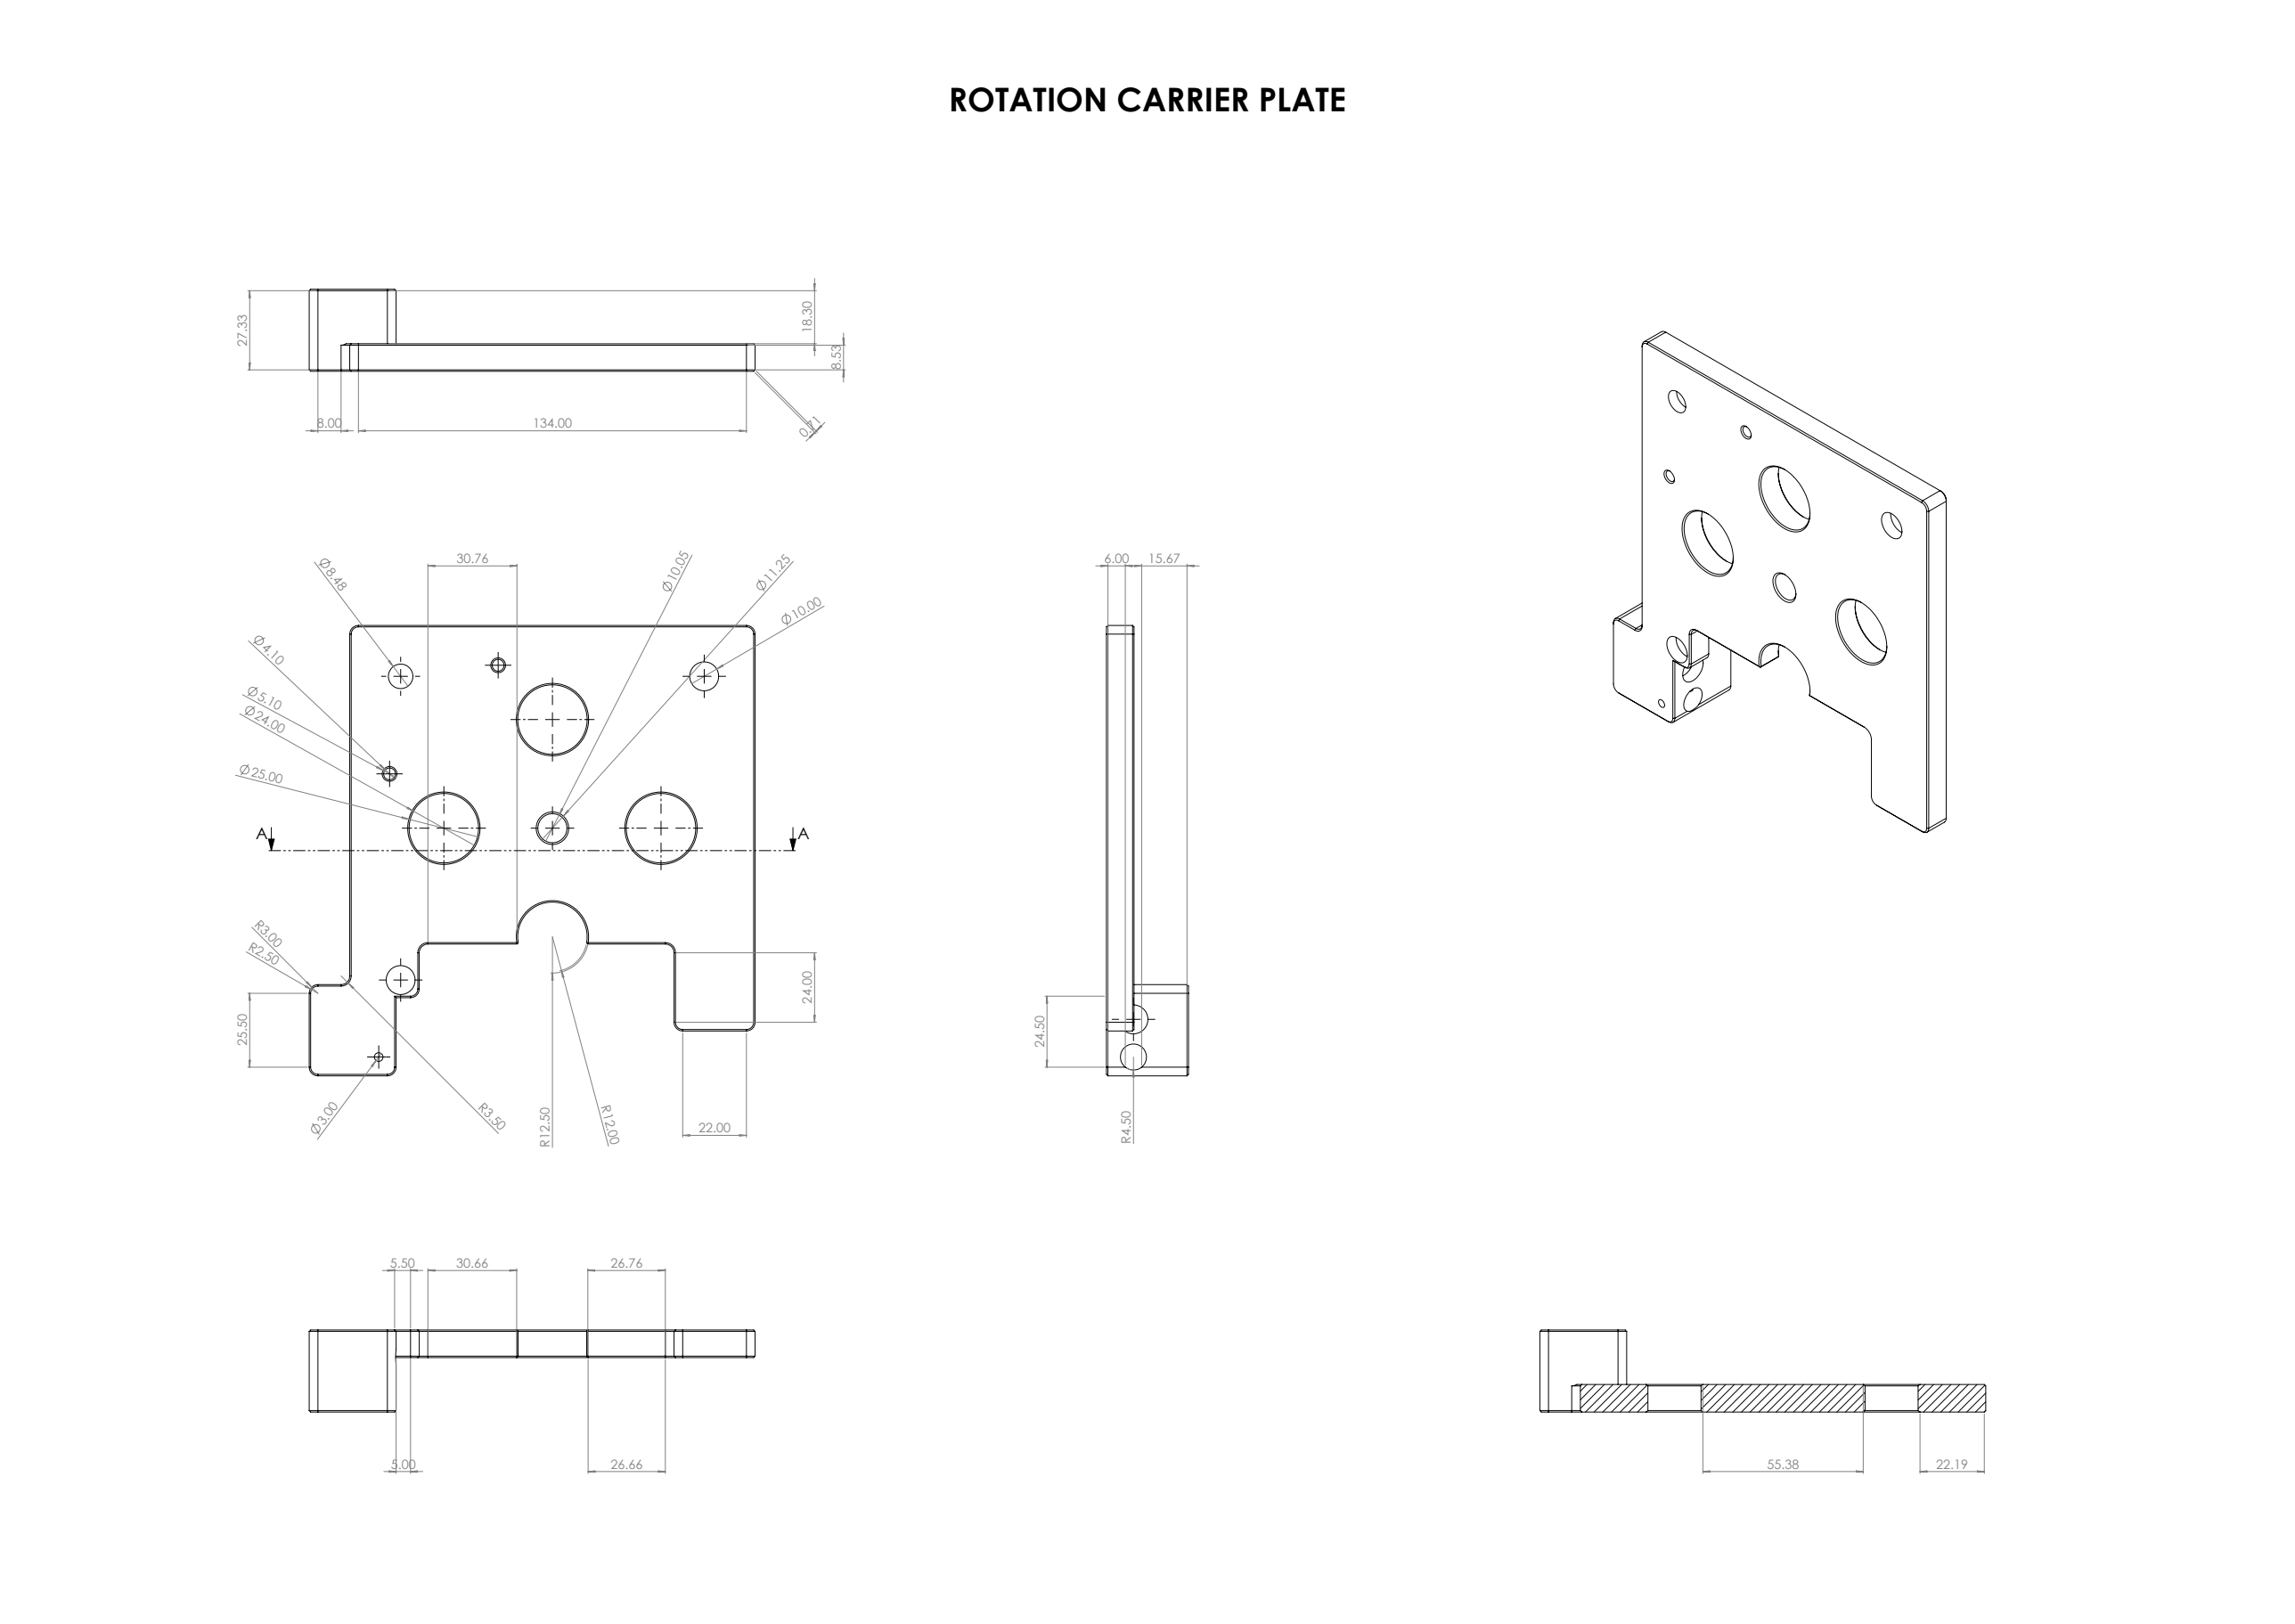
ISO-10303-21;
HEADER;
/* Generated by software containing ST-Developer
 * from STEP Tools, Inc. (www.steptools.com) 
 */

FILE_DESCRIPTION(
/* description */ (''),
/* implementation_level */ '2;1');

FILE_NAME(
/* name */ '02_Rotation_Carrier_Plate.step',
/* time_stamp */ '2026-10-21T01:56:51-07:00',
/* author */ (''),
/* organization */ (''),
/* preprocessor_version */ 'ST-DEVELOPER v20.2',
/* originating_system */ 'Autodesk Translation Framework v15.15.0.0',
/* authorisation */ '');

FILE_SCHEMA (('AUTOMOTIVE_DESIGN { 1 0 10303 214 3 1 1 }'));
ENDSEC;

DATA;
#10=MECHANICAL_DESIGN_GEOMETRIC_PRESENTATION_REPRESENTATION('',(#271),#82384);
#162=(
BOUNDED_CURVE()
B_SPLINE_CURVE(2,(#43228,#43229,#43230),.UNSPECIFIED.,.F.,.F.)
B_SPLINE_CURVE_WITH_KNOTS((3,3),(0.0459620214738357,0.0928848613146929),
 .UNSPECIFIED.)
CURVE()
GEOMETRIC_REPRESENTATION_ITEM()
RATIONAL_B_SPLINE_CURVE((1.,1.,1.))
REPRESENTATION_ITEM('')
);
#163=(
BOUNDED_CURVE()
B_SPLINE_CURVE(2,(#43236,#43237,#43238),.UNSPECIFIED.,.F.,.F.)
B_SPLINE_CURVE_WITH_KNOTS((3,3),(0.,0.040804494448543),.UNSPECIFIED.)
CURVE()
GEOMETRIC_REPRESENTATION_ITEM()
RATIONAL_B_SPLINE_CURVE((1.,1.0001754834699,1.00017645997855))
REPRESENTATION_ITEM('')
);
#164=(
BOUNDED_CURVE()
B_SPLINE_CURVE(2,(#43242,#43243,#43244),.UNSPECIFIED.,.F.,.F.)
B_SPLINE_CURVE_WITH_KNOTS((3,3),(0.0412611632307347,0.0820656576920018),
 .UNSPECIFIED.)
CURVE()
GEOMETRIC_REPRESENTATION_ITEM()
RATIONAL_B_SPLINE_CURVE((1.00017645997855,1.00017548346996,1.))
REPRESENTATION_ITEM('')
);
#165=(
BOUNDED_CURVE()
B_SPLINE_CURVE(2,(#43257,#43258,#43259),.UNSPECIFIED.,.F.,.F.)
B_SPLINE_CURVE_WITH_KNOTS((3,3),(2.77288184399903,2.88132188410877),
 .UNSPECIFIED.)
CURVE()
GEOMETRIC_REPRESENTATION_ITEM()
RATIONAL_B_SPLINE_CURVE((1.00662865875794,1.0034439439933,1.))
REPRESENTATION_ITEM('')
);
#166=(
BOUNDED_CURVE()
B_SPLINE_CURVE(2,(#43294,#43295,#43296),.UNSPECIFIED.,.F.,.F.)
B_SPLINE_CURVE_WITH_KNOTS((3,3),(0.0225541082777549,0.04593400953422),
 .UNSPECIFIED.)
CURVE()
GEOMETRIC_REPRESENTATION_ITEM()
RATIONAL_B_SPLINE_CURVE((1.01228995969815,1.01859260314039,1.02475566063204))
REPRESENTATION_ITEM('')
);
#167=(
BOUNDED_CURVE()
B_SPLINE_CURVE(2,(#43300,#43301,#43302),.UNSPECIFIED.,.F.,.F.)
B_SPLINE_CURVE_WITH_KNOTS((3,3),(0.,0.0469228395759985),.UNSPECIFIED.)
CURVE()
GEOMETRIC_REPRESENTATION_ITEM()
RATIONAL_B_SPLINE_CURVE((1.,1.,1.))
REPRESENTATION_ITEM('')
);
#168=(
BOUNDED_CURVE()
B_SPLINE_CURVE(2,(#43425,#43426,#43427),.UNSPECIFIED.,.F.,.F.)
B_SPLINE_CURVE_WITH_KNOTS((3,3),(0.188460067452875,0.376920134905751),
 .UNSPECIFIED.)
CURVE()
GEOMETRIC_REPRESENTATION_ITEM()
RATIONAL_B_SPLINE_CURVE((1.,1.04083299973288,1.))
REPRESENTATION_ITEM('')
);
#233=SHAPE_REPRESENTATION_RELATIONSHIP('SRR','None',#82467,#252);
#252=ADVANCED_BREP_SHAPE_REPRESENTATION('',(#290),#82366);
#271=STYLED_ITEM('',(#82617),#290);
#290=MANIFOLD_SOLID_BREP('Body1',#30662);
#457=CYLINDRICAL_SURFACE('',#31148,2.05);
#458=CYLINDRICAL_SURFACE('',#31152,2.05);
#459=CYLINDRICAL_SURFACE('',#31178,3.);
#460=CYLINDRICAL_SURFACE('',#31180,12.);
#461=CYLINDRICAL_SURFACE('',#31197,12.);
#462=CYLINDRICAL_SURFACE('',#31201,12.);
#463=CYLINDRICAL_SURFACE('',#31205,12.);
#464=CYLINDRICAL_SURFACE('',#31241,3.);
#465=CYLINDRICAL_SURFACE('',#31244,3.);
#466=CYLINDRICAL_SURFACE('',#31277,3.);
#467=CYLINDRICAL_SURFACE('',#31279,3.);
#468=CYLINDRICAL_SURFACE('',#31281,3.);
#469=CYLINDRICAL_SURFACE('',#31283,3.);
#470=CYLINDRICAL_SURFACE('',#31285,3.);
#471=CYLINDRICAL_SURFACE('',#31287,3.);
#472=CYLINDRICAL_SURFACE('',#31289,3.);
#473=CYLINDRICAL_SURFACE('',#31296,5.025);
#474=CYLINDRICAL_SURFACE('',#31297,1.5);
#475=CYLINDRICAL_SURFACE('',#31298,1.5);
#476=CYLINDRICAL_SURFACE('',#31301,4.5);
#477=CYLINDRICAL_SURFACE('',#31304,5.);
#478=CYLINDRICAL_SURFACE('',#31309,4.2379);
#479=CYLINDRICAL_SURFACE('',#31312,5.);
#480=CYLINDRICAL_SURFACE('',#31315,5.);
#481=CYLINDRICAL_SURFACE('',#31318,3.);
#482=CYLINDRICAL_SURFACE('',#31320,3.);
#1111=CIRCLE('',#31124,2.55);
#1112=CIRCLE('',#31125,2.05);
#1113=CIRCLE('',#31127,2.5);
#1114=CIRCLE('',#31128,3.5);
#1115=CIRCLE('',#31129,12.5);
#1116=CIRCLE('',#31130,3.5);
#1117=CIRCLE('',#31131,2.5);
#1118=CIRCLE('',#31132,2.5);
#1119=CIRCLE('',#31133,2.5);
#1120=CIRCLE('',#31134,2.5);
#1121=CIRCLE('',#31135,3.5);
#1122=CIRCLE('',#31136,2.5);
#1123=CIRCLE('',#31137,2.5);
#1124=CIRCLE('',#31138,2.50000000000001);
#1125=CIRCLE('',#31139,2.55);
#1126=CIRCLE('',#31140,12.5);
#1127=CIRCLE('',#31141,12.5);
#1128=CIRCLE('',#31142,1.5);
#1129=CIRCLE('',#31143,5.);
#1130=CIRCLE('',#31144,5.);
#1131=CIRCLE('',#31145,4.2379);
#1132=CIRCLE('',#31146,5.625);
#1133=CIRCLE('',#31147,12.5);
#1134=CIRCLE('',#31149,2.05);
#1135=CIRCLE('',#31151,2.05);
#1136=CIRCLE('',#31153,2.05);
#1137=CIRCLE('',#31156,3.);
#1138=CIRCLE('',#31159,3.);
#1139=CIRCLE('',#31162,12.);
#1140=CIRCLE('',#31167,3.);
#1141=CIRCLE('',#31168,2.5);
#1142=CIRCLE('',#31171,3.);
#1143=CIRCLE('',#31172,3.5);
#1144=CIRCLE('',#31175,12.);
#1145=CIRCLE('',#31176,12.5);
#1146=CIRCLE('',#31184,12.5);
#1147=CIRCLE('',#31185,12.);
#1148=CIRCLE('',#31187,3.);
#1149=CIRCLE('',#31188,3.5);
#1150=CIRCLE('',#31189,2.5);
#1151=CIRCLE('',#31190,2.5);
#1152=CIRCLE('',#31191,2.5);
#1153=CIRCLE('',#31192,2.5);
#1154=CIRCLE('',#31193,3.5);
#1155=CIRCLE('',#31194,12.5);
#1156=CIRCLE('',#31195,5.025);
#1157=CIRCLE('',#31196,12.5);
#1158=CIRCLE('',#31198,12.);
#1159=CIRCLE('',#31200,12.);
#1160=CIRCLE('',#31202,12.);
#1161=CIRCLE('',#31204,12.);
#1162=CIRCLE('',#31206,12.);
#1163=CIRCLE('',#31208,3.);
#1164=CIRCLE('',#31211,3.);
#1165=CIRCLE('',#31214,3.);
#1166=CIRCLE('',#31217,3.);
#1167=CIRCLE('',#31220,3.);
#1168=CIRCLE('',#31223,3.);
#1169=CIRCLE('',#31227,3.);
#1170=CIRCLE('',#31228,2.5);
#1171=CIRCLE('',#31231,3.);
#1172=CIRCLE('',#31232,2.5);
#1173=CIRCLE('',#31235,3.);
#1174=CIRCLE('',#31236,2.5);
#1175=CIRCLE('',#31239,3.);
#1176=CIRCLE('',#31240,2.50000000000001);
#1177=CIRCLE('',#31242,3.);
#1178=CIRCLE('',#31245,3.);
#1179=CIRCLE('',#31247,4.5);
#1180=CIRCLE('',#31248,4.5);
#1181=CIRCLE('',#31249,5.);
#1182=CIRCLE('',#31252,3.);
#1183=CIRCLE('',#31255,3.);
#1184=CIRCLE('',#31258,3.);
#1185=CIRCLE('',#31261,3.);
#1186=CIRCLE('',#31264,3.);
#1187=CIRCLE('',#31267,3.);
#1188=CIRCLE('',#31270,3.);
#1189=CIRCLE('',#31295,5.025);
#1190=CIRCLE('',#31299,1.5);
#1191=CIRCLE('',#31302,4.5);
#1192=CIRCLE('',#31305,5.);
#1193=CIRCLE('',#31310,4.2379);
#1194=CIRCLE('',#31313,5.);
#1195=CIRCLE('',#31316,5.);
#1899=CONICAL_SURFACE('',#31123,2.3,0.785398163397448);
#1900=CONICAL_SURFACE('',#31150,2.3,0.785398163397451);
#1901=CONICAL_SURFACE('',#31155,2.75,0.785398163397449);
#1902=CONICAL_SURFACE('',#31158,3.25,0.785398163397449);
#1903=CONICAL_SURFACE('',#31161,12.25,0.785398163397448);
#1904=CONICAL_SURFACE('',#31166,2.75,0.785398163397449);
#1905=CONICAL_SURFACE('',#31170,3.25,0.785398163397449);
#1906=CONICAL_SURFACE('',#31174,12.25,0.785398163397455);
#1907=CONICAL_SURFACE('',#31183,12.25,0.785398163397451);
#1908=CONICAL_SURFACE('',#31199,12.25,0.785398163397448);
#1909=CONICAL_SURFACE('',#31203,12.25,0.785398163397448);
#1910=CONICAL_SURFACE('',#31207,3.25,0.785398163397448);
#1911=CONICAL_SURFACE('',#31210,2.75,0.785398163397449);
#1912=CONICAL_SURFACE('',#31213,2.75,0.785398163397449);
#1913=CONICAL_SURFACE('',#31216,2.75,0.785398163397449);
#1914=CONICAL_SURFACE('',#31219,2.75,0.785398163397449);
#1915=CONICAL_SURFACE('',#31222,3.25,0.785398163397448);
#1916=CONICAL_SURFACE('',#31226,2.75,0.785398163397448);
#1917=CONICAL_SURFACE('',#31230,2.75,0.785398163397447);
#1918=CONICAL_SURFACE('',#31234,2.75,0.785398163397447);
#1919=CONICAL_SURFACE('',#31238,2.75,0.785398163397443);
#1920=CONICAL_SURFACE('',#31251,3.25,0.785398163397448);
#1921=CONICAL_SURFACE('',#31254,2.75,0.785398163397449);
#1922=CONICAL_SURFACE('',#31257,2.75,0.785398163397449);
#1923=CONICAL_SURFACE('',#31260,2.75,0.785398163397449);
#1924=CONICAL_SURFACE('',#31263,2.75,0.785398163397449);
#1925=CONICAL_SURFACE('',#31266,3.25,0.785398163397448);
#1926=CONICAL_SURFACE('',#31269,2.75,0.785398163397449);
#1927=CONICAL_SURFACE('',#31272,2.75,0.785398163397449);
#1928=CONICAL_SURFACE('',#31274,2.75,0.785398163397443);
#1929=CONICAL_SURFACE('',#31291,12.25,0.785398163397448);
#1930=CONICAL_SURFACE('',#31292,12.25,0.785398163397448);
#1931=CONICAL_SURFACE('',#31293,12.25,0.785398163397451);
#1932=CONICAL_SURFACE('',#31294,5.325,0.785398163397447);
#2303=B_SPLINE_CURVE_WITH_KNOTS('',3,(#43245,#43246,#43247,#43248),
 .UNSPECIFIED.,.F.,.F.,(4,4),(0.,0.0472495496003301),.UNSPECIFIED.);
#2304=B_SPLINE_CURVE_WITH_KNOTS('',3,(#43495,#43496,#43497,#43498,#43499,
#43500,#43501,#43502,#43503,#43504),.UNSPECIFIED.,.F.,.F.,(4,2,2,2,4),(0.495600103897638,
0.617811944958686,0.790142329574639,0.962472714190591,1.08468455525164),
 .UNSPECIFIED.);
#2305=B_SPLINE_CURVE_WITH_KNOTS('',3,(#43626,#43627,#43628,#43629,#43630,
#43631,#43632,#43633,#43634,#43635,#43636,#43637,#43638,#43639,#43640,#43641,
#43642,#43643),.UNSPECIFIED.,.F.,.F.,(4,2,2,2,2,2,2,2,4),(0.227910044047723,
0.284874338888031,0.34183863372834,0.398829360911893,0.455820088095446,
0.512810815278999,0.569801542462552,0.626765837302861,0.683730132143169),
 .UNSPECIFIED.);
#2306=B_SPLINE_CURVE_WITH_KNOTS('',3,(#43645,#43646,#43647,#43648,#43649,
#43650,#43651,#43652,#43653,#43654),.UNSPECIFIED.,.F.,.F.,(4,2,2,2,4),(0.,
0.0569907271835534,0.113981454367107,0.170945749207415,0.227910044047723),
 .UNSPECIFIED.);
#2307=B_SPLINE_CURVE_WITH_KNOTS('',3,(#43655,#43656,#43657,#43658,#43659,
#43660,#43661,#43662,#43663,#43664),.UNSPECIFIED.,.F.,.F.,(4,2,2,2,4),(0.683730132143169,
0.740694426983477,0.797658721823785,0.854649449007338,0.911640176190892),
 .UNSPECIFIED.);
#2308=B_SPLINE_CURVE_WITH_KNOTS('',3,(#43668,#43669,#43670,#43671,#43672,
#43673,#43674,#43675,#43676,#43677),.UNSPECIFIED.,.F.,.F.,(4,2,2,2,4),(0.,
0.0569907271835534,0.113981454367107,0.170945749207415,0.227910044047723),
 .UNSPECIFIED.);
#2309=B_SPLINE_CURVE_WITH_KNOTS('',3,(#43678,#43679,#43680,#43681,#43682,
#43683,#43684,#43685,#43686,#43687,#43688,#43689,#43690,#43691,#43692,#43693,
#43694,#43695,#43696,#43697,#43698,#43699,#43700,#43701,#43702,#43703),
 .UNSPECIFIED.,.F.,.F.,(4,2,2,2,2,2,2,2,2,2,2,2,4),(0.227910044047723,0.284874338888031,
0.34183863372834,0.398829360911893,0.455820088095446,0.512810815278999,
0.569801542462552,0.626765837302861,0.683730132143169,0.740694426983477,
0.797658721823785,0.854649449007338,0.911640176190892),.UNSPECIFIED.);
#3321=FACE_BOUND('',#5637,.T.);
#3322=FACE_BOUND('',#5638,.T.);
#3323=FACE_BOUND('',#5639,.T.);
#3324=FACE_BOUND('',#5640,.T.);
#3325=FACE_BOUND('',#5641,.T.);
#3326=FACE_BOUND('',#5642,.T.);
#3327=FACE_BOUND('',#5643,.T.);
#3328=FACE_BOUND('',#5644,.T.);
#3329=FACE_BOUND('',#5645,.T.);
#3330=FACE_BOUND('',#5646,.T.);
#3331=FACE_BOUND('',#5672,.T.);
#3332=FACE_BOUND('',#5673,.T.);
#3333=FACE_BOUND('',#5674,.T.);
#3334=FACE_BOUND('',#5675,.T.);
#3335=FACE_BOUND('',#5705,.T.);
#3336=FACE_BOUND('',#5749,.T.);
#3842=FACE_OUTER_BOUND('',#5635,.T.);
#3843=FACE_OUTER_BOUND('',#5636,.T.);
#3844=FACE_OUTER_BOUND('',#5647,.T.);
#3845=FACE_OUTER_BOUND('',#5648,.T.);
#3846=FACE_OUTER_BOUND('',#5649,.T.);
#3847=FACE_OUTER_BOUND('',#5650,.T.);
#3848=FACE_OUTER_BOUND('',#5651,.T.);
#3849=FACE_OUTER_BOUND('',#5652,.T.);
#3850=FACE_OUTER_BOUND('',#5653,.T.);
#3851=FACE_OUTER_BOUND('',#5654,.T.);
#3852=FACE_OUTER_BOUND('',#5655,.T.);
#3853=FACE_OUTER_BOUND('',#5656,.T.);
#3854=FACE_OUTER_BOUND('',#5657,.T.);
#3855=FACE_OUTER_BOUND('',#5658,.T.);
#3856=FACE_OUTER_BOUND('',#5659,.T.);
#3857=FACE_OUTER_BOUND('',#5660,.T.);
#3858=FACE_OUTER_BOUND('',#5661,.T.);
#3859=FACE_OUTER_BOUND('',#5662,.T.);
#3860=FACE_OUTER_BOUND('',#5663,.T.);
#3861=FACE_OUTER_BOUND('',#5664,.T.);
#3862=FACE_OUTER_BOUND('',#5665,.T.);
#3863=FACE_OUTER_BOUND('',#5666,.T.);
#3864=FACE_OUTER_BOUND('',#5667,.T.);
#3865=FACE_OUTER_BOUND('',#5668,.T.);
#3866=FACE_OUTER_BOUND('',#5669,.T.);
#3867=FACE_OUTER_BOUND('',#5670,.T.);
#3868=FACE_OUTER_BOUND('',#5671,.T.);
#3869=FACE_OUTER_BOUND('',#5676,.T.);
#3870=FACE_OUTER_BOUND('',#5677,.T.);
#3871=FACE_OUTER_BOUND('',#5678,.T.);
#3872=FACE_OUTER_BOUND('',#5679,.T.);
#3873=FACE_OUTER_BOUND('',#5680,.T.);
#3874=FACE_OUTER_BOUND('',#5681,.T.);
#3875=FACE_OUTER_BOUND('',#5682,.T.);
#3876=FACE_OUTER_BOUND('',#5683,.T.);
#3877=FACE_OUTER_BOUND('',#5684,.T.);
#3878=FACE_OUTER_BOUND('',#5685,.T.);
#3879=FACE_OUTER_BOUND('',#5686,.T.);
#3880=FACE_OUTER_BOUND('',#5687,.T.);
#3881=FACE_OUTER_BOUND('',#5688,.T.);
#3882=FACE_OUTER_BOUND('',#5689,.T.);
#3883=FACE_OUTER_BOUND('',#5690,.T.);
#3884=FACE_OUTER_BOUND('',#5691,.T.);
#3885=FACE_OUTER_BOUND('',#5692,.T.);
#3886=FACE_OUTER_BOUND('',#5693,.T.);
#3887=FACE_OUTER_BOUND('',#5694,.T.);
#3888=FACE_OUTER_BOUND('',#5695,.T.);
#3889=FACE_OUTER_BOUND('',#5696,.T.);
#3890=FACE_OUTER_BOUND('',#5697,.T.);
#3891=FACE_OUTER_BOUND('',#5698,.T.);
#3892=FACE_OUTER_BOUND('',#5699,.T.);
#3893=FACE_OUTER_BOUND('',#5700,.T.);
#3894=FACE_OUTER_BOUND('',#5701,.T.);
#3895=FACE_OUTER_BOUND('',#5702,.T.);
#3896=FACE_OUTER_BOUND('',#5703,.T.);
#3897=FACE_OUTER_BOUND('',#5704,.T.);
#3898=FACE_OUTER_BOUND('',#5706,.T.);
#3899=FACE_OUTER_BOUND('',#5707,.T.);
#3900=FACE_OUTER_BOUND('',#5708,.T.);
#3901=FACE_OUTER_BOUND('',#5709,.T.);
#3902=FACE_OUTER_BOUND('',#5710,.T.);
#3903=FACE_OUTER_BOUND('',#5711,.T.);
#3904=FACE_OUTER_BOUND('',#5712,.T.);
#3905=FACE_OUTER_BOUND('',#5713,.T.);
#3906=FACE_OUTER_BOUND('',#5714,.T.);
#3907=FACE_OUTER_BOUND('',#5715,.T.);
#3908=FACE_OUTER_BOUND('',#5716,.T.);
#3909=FACE_OUTER_BOUND('',#5717,.T.);
#3910=FACE_OUTER_BOUND('',#5718,.T.);
#3911=FACE_OUTER_BOUND('',#5719,.T.);
#3912=FACE_OUTER_BOUND('',#5720,.T.);
#3913=FACE_OUTER_BOUND('',#5721,.T.);
#3914=FACE_OUTER_BOUND('',#5722,.T.);
#3915=FACE_OUTER_BOUND('',#5723,.T.);
#3916=FACE_OUTER_BOUND('',#5724,.T.);
#3917=FACE_OUTER_BOUND('',#5725,.T.);
#3918=FACE_OUTER_BOUND('',#5726,.T.);
#3919=FACE_OUTER_BOUND('',#5727,.T.);
#3920=FACE_OUTER_BOUND('',#5728,.T.);
#3921=FACE_OUTER_BOUND('',#5729,.T.);
#3922=FACE_OUTER_BOUND('',#5730,.T.);
#3923=FACE_OUTER_BOUND('',#5731,.T.);
#3924=FACE_OUTER_BOUND('',#5732,.T.);
#3925=FACE_OUTER_BOUND('',#5733,.T.);
#3926=FACE_OUTER_BOUND('',#5734,.T.);
#3927=FACE_OUTER_BOUND('',#5735,.T.);
#3928=FACE_OUTER_BOUND('',#5736,.T.);
#3929=FACE_OUTER_BOUND('',#5737,.T.);
#3930=FACE_OUTER_BOUND('',#5738,.T.);
#3931=FACE_OUTER_BOUND('',#5739,.T.);
#3932=FACE_OUTER_BOUND('',#5740,.T.);
#3933=FACE_OUTER_BOUND('',#5741,.T.);
#3934=FACE_OUTER_BOUND('',#5742,.T.);
#3935=FACE_OUTER_BOUND('',#5743,.T.);
#3936=FACE_OUTER_BOUND('',#5744,.T.);
#3937=FACE_OUTER_BOUND('',#5745,.T.);
#3938=FACE_OUTER_BOUND('',#5746,.T.);
#3939=FACE_OUTER_BOUND('',#5747,.T.);
#3940=FACE_OUTER_BOUND('',#5748,.T.);
#3941=FACE_OUTER_BOUND('',#5750,.T.);
#3942=FACE_OUTER_BOUND('',#5751,.T.);
#3943=FACE_OUTER_BOUND('',#5752,.T.);
#3944=FACE_OUTER_BOUND('',#5753,.T.);
#3945=FACE_OUTER_BOUND('',#5754,.T.);
#3946=FACE_OUTER_BOUND('',#5755,.T.);
#3947=FACE_OUTER_BOUND('',#5756,.T.);
#3948=FACE_OUTER_BOUND('',#5757,.T.);
#3949=FACE_OUTER_BOUND('',#5758,.T.);
#3950=FACE_OUTER_BOUND('',#5759,.T.);
#3951=FACE_OUTER_BOUND('',#5760,.T.);
#3952=FACE_OUTER_BOUND('',#5761,.T.);
#3953=FACE_OUTER_BOUND('',#5762,.T.);
#3954=FACE_OUTER_BOUND('',#5763,.T.);
#5635=EDGE_LOOP('',(#20603,#20604,#20605,#20606));
#5636=EDGE_LOOP('',(#20607,#20608,#20609,#20610,#20611,#20612,#20613,#20614,
#20615,#20616,#20617,#20618,#20619,#20620,#20621,#20622,#20623,#20624,#20625,
#20626,#20627,#20628,#20629,#20630,#20631));
#5637=EDGE_LOOP('',(#20632));
#5638=EDGE_LOOP('',(#20633));
#5639=EDGE_LOOP('',(#20634));
#5640=EDGE_LOOP('',(#20635));
#5641=EDGE_LOOP('',(#20636));
#5642=EDGE_LOOP('',(#20637));
#5643=EDGE_LOOP('',(#20638));
#5644=EDGE_LOOP('',(#20639));
#5645=EDGE_LOOP('',(#20640));
#5646=EDGE_LOOP('',(#20641));
#5647=EDGE_LOOP('',(#20642,#20643,#20644,#20645));
#5648=EDGE_LOOP('',(#20646,#20647,#20648,#20649));
#5649=EDGE_LOOP('',(#20650,#20651,#20652,#20653));
#5650=EDGE_LOOP('',(#20654,#20655,#20656,#20657));
#5651=EDGE_LOOP('',(#20658,#20659,#20660,#20661));
#5652=EDGE_LOOP('',(#20662,#20663,#20664,#20665));
#5653=EDGE_LOOP('',(#20666,#20667,#20668,#20669));
#5654=EDGE_LOOP('',(#20670,#20671,#20672,#20673,#20674));
#5655=EDGE_LOOP('',(#20675,#20676,#20677,#20678,#20679,#20680));
#5656=EDGE_LOOP('',(#20681,#20682,#20683,#20684,#20685));
#5657=EDGE_LOOP('',(#20686,#20687,#20688));
#5658=EDGE_LOOP('',(#20689,#20690,#20691,#20692));
#5659=EDGE_LOOP('',(#20693,#20694,#20695,#20696));
#5660=EDGE_LOOP('',(#20697,#20698,#20699,#20700));
#5661=EDGE_LOOP('',(#20701,#20702,#20703,#20704));
#5662=EDGE_LOOP('',(#20705,#20706,#20707,#20708));
#5663=EDGE_LOOP('',(#20709,#20710,#20711,#20712,#20713));
#5664=EDGE_LOOP('',(#20714,#20715,#20716,#20717));
#5665=EDGE_LOOP('',(#20718,#20719,#20720,#20721));
#5666=EDGE_LOOP('',(#20722,#20723,#20724,#20725));
#5667=EDGE_LOOP('',(#20726,#20727,#20728,#20729));
#5668=EDGE_LOOP('',(#20730,#20731,#20732,#20733,#20734,#20735));
#5669=EDGE_LOOP('',(#20736,#20737,#20738,#20739,#20740));
#5670=EDGE_LOOP('',(#20741,#20742,#20743,#20744));
#5671=EDGE_LOOP('',(#20745,#20746,#20747,#20748,#20749,#20750,#20751,#20752,
#20753,#20754,#20755,#20756,#20757,#20758,#20759,#20760,#20761,#20762,#20763,
#20764,#20765));
#5672=EDGE_LOOP('',(#20766));
#5673=EDGE_LOOP('',(#20767));
#5674=EDGE_LOOP('',(#20768));
#5675=EDGE_LOOP('',(#20769));
#5676=EDGE_LOOP('',(#20770,#20771,#20772,#20773));
#5677=EDGE_LOOP('',(#20774,#20775,#20776,#20777));
#5678=EDGE_LOOP('',(#20778,#20779,#20780,#20781));
#5679=EDGE_LOOP('',(#20782,#20783,#20784,#20785));
#5680=EDGE_LOOP('',(#20786,#20787,#20788,#20789));
#5681=EDGE_LOOP('',(#20790,#20791,#20792,#20793));
#5682=EDGE_LOOP('',(#20794,#20795,#20796,#20797));
#5683=EDGE_LOOP('',(#20798,#20799,#20800,#20801));
#5684=EDGE_LOOP('',(#20802,#20803,#20804,#20805));
#5685=EDGE_LOOP('',(#20806,#20807,#20808,#20809));
#5686=EDGE_LOOP('',(#20810,#20811,#20812,#20813));
#5687=EDGE_LOOP('',(#20814,#20815,#20816,#20817));
#5688=EDGE_LOOP('',(#20818,#20819,#20820,#20821));
#5689=EDGE_LOOP('',(#20822,#20823,#20824,#20825));
#5690=EDGE_LOOP('',(#20826,#20827,#20828,#20829));
#5691=EDGE_LOOP('',(#20830,#20831,#20832,#20833));
#5692=EDGE_LOOP('',(#20834,#20835,#20836,#20837,#20838));
#5693=EDGE_LOOP('',(#20839,#20840,#20841,#20842));
#5694=EDGE_LOOP('',(#20843,#20844,#20845,#20846));
#5695=EDGE_LOOP('',(#20847,#20848,#20849,#20850));
#5696=EDGE_LOOP('',(#20851,#20852,#20853,#20854));
#5697=EDGE_LOOP('',(#20855,#20856,#20857,#20858));
#5698=EDGE_LOOP('',(#20859,#20860,#20861,#20862));
#5699=EDGE_LOOP('',(#20863,#20864,#20865,#20866));
#5700=EDGE_LOOP('',(#20867,#20868,#20869,#20870));
#5701=EDGE_LOOP('',(#20871,#20872,#20873,#20874));
#5702=EDGE_LOOP('',(#20875,#20876,#20877,#20878));
#5703=EDGE_LOOP('',(#20879,#20880,#20881,#20882,#20883,#20884));
#5704=EDGE_LOOP('',(#20885,#20886,#20887,#20888,#20889,#20890,#20891,#20892,
#20893,#20894));
#5705=EDGE_LOOP('',(#20895));
#5706=EDGE_LOOP('',(#20896,#20897,#20898,#20899,#20900,#20901,#20902,#20903));
#5707=EDGE_LOOP('',(#20904,#20905,#20906,#20907));
#5708=EDGE_LOOP('',(#20908,#20909,#20910,#20911));
#5709=EDGE_LOOP('',(#20912,#20913,#20914,#20915));
#5710=EDGE_LOOP('',(#20916,#20917,#20918,#20919));
#5711=EDGE_LOOP('',(#20920,#20921,#20922,#20923));
#5712=EDGE_LOOP('',(#20924,#20925,#20926,#20927));
#5713=EDGE_LOOP('',(#20928,#20929,#20930,#20931));
#5714=EDGE_LOOP('',(#20932,#20933,#20934,#20935));
#5715=EDGE_LOOP('',(#20936,#20937,#20938,#20939));
#5716=EDGE_LOOP('',(#20940,#20941,#20942,#20943));
#5717=EDGE_LOOP('',(#20944,#20945,#20946,#20947));
#5718=EDGE_LOOP('',(#20948,#20949,#20950,#20951));
#5719=EDGE_LOOP('',(#20952,#20953,#20954,#20955));
#5720=EDGE_LOOP('',(#20956,#20957,#20958,#20959));
#5721=EDGE_LOOP('',(#20960,#20961,#20962,#20963));
#5722=EDGE_LOOP('',(#20964,#20965,#20966,#20967));
#5723=EDGE_LOOP('',(#20968,#20969,#20970,#20971));
#5724=EDGE_LOOP('',(#20972,#20973,#20974,#20975));
#5725=EDGE_LOOP('',(#20976,#20977,#20978,#20979));
#5726=EDGE_LOOP('',(#20980,#20981,#20982,#20983));
#5727=EDGE_LOOP('',(#20984,#20985,#20986,#20987,#20988,#20989,#20990));
#5728=EDGE_LOOP('',(#20991,#20992,#20993,#20994));
#5729=EDGE_LOOP('',(#20995,#20996,#20997,#20998));
#5730=EDGE_LOOP('',(#20999,#21000,#21001,#21002));
#5731=EDGE_LOOP('',(#21003,#21004,#21005,#21006));
#5732=EDGE_LOOP('',(#21007,#21008,#21009,#21010));
#5733=EDGE_LOOP('',(#21011,#21012,#21013,#21014));
#5734=EDGE_LOOP('',(#21015,#21016,#21017,#21018));
#5735=EDGE_LOOP('',(#21019,#21020,#21021,#21022));
#5736=EDGE_LOOP('',(#21023,#21024,#21025,#21026));
#5737=EDGE_LOOP('',(#21027,#21028,#21029,#21030));
#5738=EDGE_LOOP('',(#21031,#21032,#21033,#21034));
#5739=EDGE_LOOP('',(#21035,#21036,#21037,#21038));
#5740=EDGE_LOOP('',(#21039,#21040,#21041,#21042));
#5741=EDGE_LOOP('',(#21043,#21044,#21045,#21046));
#5742=EDGE_LOOP('',(#21047,#21048,#21049,#21050));
#5743=EDGE_LOOP('',(#21051,#21052,#21053,#21054));
#5744=EDGE_LOOP('',(#21055,#21056,#21057,#21058));
#5745=EDGE_LOOP('',(#21059,#21060,#21061,#21062,#21063,#21064));
#5746=EDGE_LOOP('',(#21065,#21066,#21067,#21068,#21069));
#5747=EDGE_LOOP('',(#21070));
#5748=EDGE_LOOP('',(#21071,#21072,#21073,#21074,#21075,#21076,#21077,#21078,
#21079,#21080,#21081));
#5749=EDGE_LOOP('',(#21082,#21083));
#5750=EDGE_LOOP('',(#21084));
#5751=EDGE_LOOP('',(#21085,#21086,#21087,#21088));
#5752=EDGE_LOOP('',(#21089));
#5753=EDGE_LOOP('',(#21090));
#5754=EDGE_LOOP('',(#21091));
#5755=EDGE_LOOP('',(#21092,#21093,#21094,#21095));
#5756=EDGE_LOOP('',(#21096));
#5757=EDGE_LOOP('',(#21097,#21098,#21099,#21100));
#5758=EDGE_LOOP('',(#21101));
#5759=EDGE_LOOP('',(#21102,#21103,#21104,#21105));
#5760=EDGE_LOOP('',(#21106));
#5761=EDGE_LOOP('',(#21107,#21108,#21109,#21110));
#5762=EDGE_LOOP('',(#21111,#21112,#21113,#21114));
#5763=EDGE_LOOP('',(#21115,#21116,#21117,#21118));
#7754=LINE('',#43125,#10060);
#7755=LINE('',#43130,#10061);
#7756=LINE('',#43132,#10062);
#7757=LINE('',#43136,#10063);
#7758=LINE('',#43140,#10064);
#7759=LINE('',#43144,#10065);
#7760=LINE('',#43148,#10066);
#7761=LINE('',#43152,#10067);
#7762=LINE('',#43156,#10068);
#7763=LINE('',#43160,#10069);
#7764=LINE('',#43164,#10070);
#7765=LINE('',#43168,#10071);
#7766=LINE('',#43172,#10072);
#7767=LINE('',#43176,#10073);
#7768=LINE('',#43198,#10074);
#7769=LINE('',#43202,#10075);
#7770=LINE('',#43206,#10076);
#7771=LINE('',#43210,#10077);
#7772=LINE('',#43212,#10078);
#7773=LINE('',#43213,#10079);
#7774=LINE('',#43217,#10080);
#7775=LINE('',#43220,#10081);
#7776=LINE('',#43221,#10082);
#7777=LINE('',#43225,#10083);
#7778=LINE('',#43232,#10084);
#7779=LINE('',#43233,#10085);
#7780=LINE('',#43251,#10086);
#7781=LINE('',#43253,#10087);
#7782=LINE('',#43254,#10088);
#7783=LINE('',#43260,#10089);
#7784=LINE('',#43264,#10090);
#7785=LINE('',#43266,#10091);
#7786=LINE('',#43268,#10092);
#7787=LINE('',#43269,#10093);
#7788=LINE('',#43273,#10094);
#7789=LINE('',#43279,#10095);
#7790=LINE('',#43280,#10096);
#7791=LINE('',#43281,#10097);
#7792=LINE('',#43285,#10098);
#7793=LINE('',#43289,#10099);
#7794=LINE('',#43290,#10100);
#7795=LINE('',#43304,#10101);
#7796=LINE('',#43305,#10102);
#7797=LINE('',#43307,#10103);
#7798=LINE('',#43310,#10104);
#7799=LINE('',#43313,#10105);
#7800=LINE('',#43315,#10106);
#7801=LINE('',#43316,#10107);
#7802=LINE('',#43319,#10108);
#7803=LINE('',#43321,#10109);
#7804=LINE('',#43322,#10110);
#7805=LINE('',#43327,#10111);
#7806=LINE('',#43331,#10112);
#7807=LINE('',#43335,#10113);
#7808=LINE('',#43339,#10114);
#7809=LINE('',#43343,#10115);
#7810=LINE('',#43347,#10116);
#7811=LINE('',#43351,#10117);
#7812=LINE('',#43355,#10118);
#7813=LINE('',#43366,#10119);
#7814=LINE('',#43369,#10120);
#7815=LINE('',#43374,#10121);
#7816=LINE('',#43377,#10122);
#7817=LINE('',#43382,#10123);
#7818=LINE('',#43385,#10124);
#7819=LINE('',#43389,#10125);
#7820=LINE('',#43390,#10126);
#7821=LINE('',#43393,#10127);
#7822=LINE('',#43397,#10128);
#7823=LINE('',#43398,#10129);
#7824=LINE('',#43401,#10130);
#7825=LINE('',#43405,#10131);
#7826=LINE('',#43406,#10132);
#7827=LINE('',#43409,#10133);
#7828=LINE('',#43413,#10134);
#7829=LINE('',#43414,#10135);
#7830=LINE('',#43417,#10136);
#7831=LINE('',#43421,#10137);
#7832=LINE('',#43422,#10138);
#7833=LINE('',#43431,#10139);
#7834=LINE('',#43432,#10140);
#7835=LINE('',#43436,#10141);
#7836=LINE('',#43438,#10142);
#7837=LINE('',#43440,#10143);
#7838=LINE('',#43441,#10144);
#7839=LINE('',#43445,#10145);
#7840=LINE('',#43451,#10146);
#7841=LINE('',#43452,#10147);
#7842=LINE('',#43453,#10148);
#7843=LINE('',#43457,#10149);
#7844=LINE('',#43463,#10150);
#7845=LINE('',#43464,#10151);
#7846=LINE('',#43465,#10152);
#7847=LINE('',#43469,#10153);
#7848=LINE('',#43475,#10154);
#7849=LINE('',#43476,#10155);
#7850=LINE('',#43477,#10156);
#7851=LINE('',#43483,#10157);
#7852=LINE('',#43486,#10158);
#7853=LINE('',#43489,#10159);
#7854=LINE('',#43490,#10160);
#7855=LINE('',#43493,#10161);
#7856=LINE('',#43506,#10162);
#7857=LINE('',#43509,#10163);
#7858=LINE('',#43510,#10164);
#7859=LINE('',#43511,#10165);
#7860=LINE('',#43521,#10166);
#7861=LINE('',#43524,#10167);
#7862=LINE('',#43525,#10168);
#7863=LINE('',#43529,#10169);
#7864=LINE('',#43532,#10170);
#7865=LINE('',#43533,#10171);
#7866=LINE('',#43537,#10172);
#7867=LINE('',#43540,#10173);
#7868=LINE('',#43541,#10174);
#7869=LINE('',#43545,#10175);
#7870=LINE('',#43548,#10176);
#7871=LINE('',#43549,#10177);
#7872=LINE('',#43553,#10178);
#7873=LINE('',#43556,#10179);
#7874=LINE('',#43557,#10180);
#7875=LINE('',#43561,#10181);
#7876=LINE('',#43564,#10182);
#7877=LINE('',#43565,#10183);
#7878=LINE('',#43569,#10184);
#7879=LINE('',#43571,#10185);
#7880=LINE('',#43572,#10186);
#7881=LINE('',#43574,#10187);
#7882=LINE('',#43576,#10188);
#7883=LINE('',#43578,#10189);
#7884=LINE('',#43581,#10190);
#7885=LINE('',#43583,#10191);
#7886=LINE('',#43585,#10192);
#7887=LINE('',#43586,#10193);
#7888=LINE('',#43588,#10194);
#7889=LINE('',#43590,#10195);
#7890=LINE('',#43592,#10196);
#7891=LINE('',#43594,#10197);
#7892=LINE('',#43596,#10198);
#7893=LINE('',#43598,#10199);
#7894=LINE('',#43600,#10200);
#7895=LINE('',#43602,#10201);
#7896=LINE('',#43604,#10202);
#7897=LINE('',#43606,#10203);
#7898=LINE('',#43608,#10204);
#7899=LINE('',#43611,#10205);
#7900=LINE('',#43613,#10206);
#7901=LINE('',#43615,#10207);
#7902=LINE('',#43618,#10208);
#7903=LINE('',#43621,#10209);
#7904=LINE('',#43624,#10210);
#7905=LINE('',#43705,#10211);
#7906=LINE('',#43709,#10212);
#7907=LINE('',#43711,#10213);
#7908=LINE('',#43716,#10214);
#7909=LINE('',#43723,#10215);
#7910=LINE('',#43728,#10216);
#7911=LINE('',#43733,#10217);
#7912=LINE('',#43737,#10218);
#10060=VECTOR('',#34255,2.3);
#10061=VECTOR('',#34260,10.);
#10062=VECTOR('',#34261,10.);
#10063=VECTOR('',#34264,10.);
#10064=VECTOR('',#34267,10.);
#10065=VECTOR('',#34270,10.);
#10066=VECTOR('',#34273,10.);
#10067=VECTOR('',#34276,10.);
#10068=VECTOR('',#34279,10.);
#10069=VECTOR('',#34282,10.);
#10070=VECTOR('',#34285,10.);
#10071=VECTOR('',#34288,10.);
#10072=VECTOR('',#34291,10.);
#10073=VECTOR('',#34294,10.);
#10074=VECTOR('',#34317,2.05);
#10075=VECTOR('',#34322,2.3);
#10076=VECTOR('',#34327,2.05);
#10077=VECTOR('',#34332,10.);
#10078=VECTOR('',#34333,10.);
#10079=VECTOR('',#34334,10.);
#10080=VECTOR('',#34339,10.);
#10081=VECTOR('',#34342,10.);
#10082=VECTOR('',#34343,10.);
#10083=VECTOR('',#34348,10.);
#10084=VECTOR('',#34351,10.);
#10085=VECTOR('',#34352,10.);
#10086=VECTOR('',#34359,10.);
#10087=VECTOR('',#34360,10.);
#10088=VECTOR('',#34361,10.);
#10089=VECTOR('',#34364,10.);
#10090=VECTOR('',#34367,10.);
#10091=VECTOR('',#34368,10.);
#10092=VECTOR('',#34369,10.);
#10093=VECTOR('',#34370,10.);
#10094=VECTOR('',#34373,10.);
#10095=VECTOR('',#34380,10.);
#10096=VECTOR('',#34381,10.);
#10097=VECTOR('',#34382,10.);
#10098=VECTOR('',#34385,10.);
#10099=VECTOR('',#34392,10.);
#10100=VECTOR('',#34393,10.);
#10101=VECTOR('',#34402,10.);
#10102=VECTOR('',#34403,10.);
#10103=VECTOR('',#34406,10.);
#10104=VECTOR('',#34411,10.);
#10105=VECTOR('',#34414,10.);
#10106=VECTOR('',#34415,10.);
#10107=VECTOR('',#34416,10.);
#10108=VECTOR('',#34419,10.);
#10109=VECTOR('',#34420,10.);
#10110=VECTOR('',#34421,10.);
#10111=VECTOR('',#34426,12.25);
#10112=VECTOR('',#34431,10.);
#10113=VECTOR('',#34434,10.);
#10114=VECTOR('',#34437,10.);
#10115=VECTOR('',#34440,10.);
#10116=VECTOR('',#34443,10.);
#10117=VECTOR('',#34446,10.);
#10118=VECTOR('',#34449,10.);
#10119=VECTOR('',#34462,12.);
#10120=VECTOR('',#34465,12.25);
#10121=VECTOR('',#34472,12.);
#10122=VECTOR('',#34475,12.25);
#10123=VECTOR('',#34482,12.);
#10124=VECTOR('',#34485,10.);
#10125=VECTOR('',#34490,10.);
#10126=VECTOR('',#34491,10.);
#10127=VECTOR('',#34494,10.);
#10128=VECTOR('',#34499,10.);
#10129=VECTOR('',#34500,10.);
#10130=VECTOR('',#34503,10.);
#10131=VECTOR('',#34508,10.);
#10132=VECTOR('',#34509,10.);
#10133=VECTOR('',#34512,10.);
#10134=VECTOR('',#34517,10.);
#10135=VECTOR('',#34518,10.);
#10136=VECTOR('',#34521,10.);
#10137=VECTOR('',#34526,10.);
#10138=VECTOR('',#34527,10.);
#10139=VECTOR('',#34534,10.);
#10140=VECTOR('',#34535,10.);
#10141=VECTOR('',#34538,10.);
#10142=VECTOR('',#34539,10.);
#10143=VECTOR('',#34540,10.);
#10144=VECTOR('',#34541,10.);
#10145=VECTOR('',#34544,10.);
#10146=VECTOR('',#34551,10.);
#10147=VECTOR('',#34552,10.);
#10148=VECTOR('',#34553,10.);
#10149=VECTOR('',#34556,10.);
#10150=VECTOR('',#34563,10.);
#10151=VECTOR('',#34564,10.);
#10152=VECTOR('',#34565,10.);
#10153=VECTOR('',#34568,10.);
#10154=VECTOR('',#34575,10.);
#10155=VECTOR('',#34576,10.);
#10156=VECTOR('',#34577,10.);
#10157=VECTOR('',#34586,10.);
#10158=VECTOR('',#34589,10.);
#10159=VECTOR('',#34592,10.);
#10160=VECTOR('',#34593,10.);
#10161=VECTOR('',#34596,10.);
#10162=VECTOR('',#34597,10.);
#10163=VECTOR('',#34602,10.);
#10164=VECTOR('',#34603,10.);
#10165=VECTOR('',#34604,10.);
#10166=VECTOR('',#34617,10.);
#10167=VECTOR('',#34620,10.);
#10168=VECTOR('',#34621,10.);
#10169=VECTOR('',#34626,10.);
#10170=VECTOR('',#34629,10.);
#10171=VECTOR('',#34630,10.);
#10172=VECTOR('',#34635,10.);
#10173=VECTOR('',#34638,10.);
#10174=VECTOR('',#34639,10.);
#10175=VECTOR('',#34644,10.);
#10176=VECTOR('',#34647,10.);
#10177=VECTOR('',#34648,10.);
#10178=VECTOR('',#34653,10.);
#10179=VECTOR('',#34656,10.);
#10180=VECTOR('',#34657,10.);
#10181=VECTOR('',#34662,10.);
#10182=VECTOR('',#34665,10.);
#10183=VECTOR('',#34666,10.);
#10184=VECTOR('',#34671,10.);
#10185=VECTOR('',#34674,10.);
#10186=VECTOR('',#34675,10.);
#10187=VECTOR('',#34678,10.);
#10188=VECTOR('',#34681,10.);
#10189=VECTOR('',#34684,10.);
#10190=VECTOR('',#34689,10.);
#10191=VECTOR('',#34692,10.);
#10192=VECTOR('',#34695,10.);
#10193=VECTOR('',#34696,10.);
#10194=VECTOR('',#34699,10.);
#10195=VECTOR('',#34702,10.);
#10196=VECTOR('',#34705,10.);
#10197=VECTOR('',#34708,10.);
#10198=VECTOR('',#34711,10.);
#10199=VECTOR('',#34714,10.);
#10200=VECTOR('',#34717,10.);
#10201=VECTOR('',#34720,10.);
#10202=VECTOR('',#34723,10.);
#10203=VECTOR('',#34726,10.);
#10204=VECTOR('',#34729,10.);
#10205=VECTOR('',#34734,12.25);
#10206=VECTOR('',#34737,12.25);
#10207=VECTOR('',#34740,12.25);
#10208=VECTOR('',#34743,5.325);
#10209=VECTOR('',#34748,5.025);
#10210=VECTOR('',#34751,1.5);
#10211=VECTOR('',#34754,1.5);
#10212=VECTOR('',#34761,4.5);
#10213=VECTOR('',#34762,4.5);
#10214=VECTOR('',#34769,5.);
#10215=VECTOR('',#34780,4.2379);
#10216=VECTOR('',#34787,5.);
#10217=VECTOR('',#34794,5.);
#10218=VECTOR('',#34801,10.);
#12425=VERTEX_POINT('',#43122);
#12426=VERTEX_POINT('',#43124);
#12427=VERTEX_POINT('',#43128);
#12428=VERTEX_POINT('',#43129);
#12429=VERTEX_POINT('',#43131);
#12430=VERTEX_POINT('',#43133);
#12431=VERTEX_POINT('',#43135);
#12432=VERTEX_POINT('',#43137);
#12433=VERTEX_POINT('',#43139);
#12434=VERTEX_POINT('',#43141);
#12435=VERTEX_POINT('',#43143);
#12436=VERTEX_POINT('',#43145);
#12437=VERTEX_POINT('',#43147);
#12438=VERTEX_POINT('',#43149);
#12439=VERTEX_POINT('',#43151);
#12440=VERTEX_POINT('',#43153);
#12441=VERTEX_POINT('',#43155);
#12442=VERTEX_POINT('',#43157);
#12443=VERTEX_POINT('',#43159);
#12444=VERTEX_POINT('',#43161);
#12445=VERTEX_POINT('',#43163);
#12446=VERTEX_POINT('',#43165);
#12447=VERTEX_POINT('',#43167);
#12448=VERTEX_POINT('',#43169);
#12449=VERTEX_POINT('',#43171);
#12450=VERTEX_POINT('',#43173);
#12451=VERTEX_POINT('',#43175);
#12452=VERTEX_POINT('',#43178);
#12453=VERTEX_POINT('',#43180);
#12454=VERTEX_POINT('',#43182);
#12455=VERTEX_POINT('',#43184);
#12456=VERTEX_POINT('',#43186);
#12457=VERTEX_POINT('',#43188);
#12458=VERTEX_POINT('',#43190);
#12459=VERTEX_POINT('',#43192);
#12460=VERTEX_POINT('',#43194);
#12461=VERTEX_POINT('',#43197);
#12462=VERTEX_POINT('',#43201);
#12463=VERTEX_POINT('',#43205);
#12464=VERTEX_POINT('',#43209);
#12465=VERTEX_POINT('',#43211);
#12466=VERTEX_POINT('',#43215);
#12467=VERTEX_POINT('',#43219);
#12468=VERTEX_POINT('',#43223);
#12469=VERTEX_POINT('',#43227);
#12470=VERTEX_POINT('',#43231);
#12471=VERTEX_POINT('',#43235);
#12472=VERTEX_POINT('',#43239);
#12473=VERTEX_POINT('',#43241);
#12474=VERTEX_POINT('',#43250);
#12475=VERTEX_POINT('',#43252);
#12476=VERTEX_POINT('',#43256);
#12477=VERTEX_POINT('',#43262);
#12478=VERTEX_POINT('',#43263);
#12479=VERTEX_POINT('',#43265);
#12480=VERTEX_POINT('',#43267);
#12481=VERTEX_POINT('',#43271);
#12482=VERTEX_POINT('',#43272);
#12483=VERTEX_POINT('',#43277);
#12484=VERTEX_POINT('',#43278);
#12485=VERTEX_POINT('',#43283);
#12486=VERTEX_POINT('',#43284);
#12487=VERTEX_POINT('',#43292);
#12488=VERTEX_POINT('',#43293);
#12489=VERTEX_POINT('',#43298);
#12490=VERTEX_POINT('',#43312);
#12491=VERTEX_POINT('',#43314);
#12492=VERTEX_POINT('',#43318);
#12493=VERTEX_POINT('',#43320);
#12494=VERTEX_POINT('',#43324);
#12495=VERTEX_POINT('',#43326);
#12496=VERTEX_POINT('',#43330);
#12497=VERTEX_POINT('',#43332);
#12498=VERTEX_POINT('',#43334);
#12499=VERTEX_POINT('',#43336);
#12500=VERTEX_POINT('',#43338);
#12501=VERTEX_POINT('',#43340);
#12502=VERTEX_POINT('',#43342);
#12503=VERTEX_POINT('',#43344);
#12504=VERTEX_POINT('',#43346);
#12505=VERTEX_POINT('',#43348);
#12506=VERTEX_POINT('',#43350);
#12507=VERTEX_POINT('',#43352);
#12508=VERTEX_POINT('',#43354);
#12509=VERTEX_POINT('',#43357);
#12510=VERTEX_POINT('',#43359);
#12511=VERTEX_POINT('',#43361);
#12512=VERTEX_POINT('',#43364);
#12513=VERTEX_POINT('',#43368);
#12514=VERTEX_POINT('',#43372);
#12515=VERTEX_POINT('',#43376);
#12516=VERTEX_POINT('',#43380);
#12517=VERTEX_POINT('',#43384);
#12518=VERTEX_POINT('',#43388);
#12519=VERTEX_POINT('',#43392);
#12520=VERTEX_POINT('',#43396);
#12521=VERTEX_POINT('',#43400);
#12522=VERTEX_POINT('',#43404);
#12523=VERTEX_POINT('',#43408);
#12524=VERTEX_POINT('',#43412);
#12525=VERTEX_POINT('',#43416);
#12526=VERTEX_POINT('',#43420);
#12527=VERTEX_POINT('',#43424);
#12528=VERTEX_POINT('',#43430);
#12529=VERTEX_POINT('',#43434);
#12530=VERTEX_POINT('',#43435);
#12531=VERTEX_POINT('',#43437);
#12532=VERTEX_POINT('',#43439);
#12533=VERTEX_POINT('',#43443);
#12534=VERTEX_POINT('',#43444);
#12535=VERTEX_POINT('',#43449);
#12536=VERTEX_POINT('',#43450);
#12537=VERTEX_POINT('',#43455);
#12538=VERTEX_POINT('',#43456);
#12539=VERTEX_POINT('',#43461);
#12540=VERTEX_POINT('',#43462);
#12541=VERTEX_POINT('',#43467);
#12542=VERTEX_POINT('',#43468);
#12543=VERTEX_POINT('',#43473);
#12544=VERTEX_POINT('',#43474);
#12545=VERTEX_POINT('',#43482);
#12546=VERTEX_POINT('',#43484);
#12547=VERTEX_POINT('',#43488);
#12548=VERTEX_POINT('',#43492);
#12549=VERTEX_POINT('',#43494);
#12550=VERTEX_POINT('',#43505);
#12551=VERTEX_POINT('',#43512);
#12552=VERTEX_POINT('',#43515);
#12553=VERTEX_POINT('',#43519);
#12554=VERTEX_POINT('',#43523);
#12555=VERTEX_POINT('',#43527);
#12556=VERTEX_POINT('',#43531);
#12557=VERTEX_POINT('',#43535);
#12558=VERTEX_POINT('',#43539);
#12559=VERTEX_POINT('',#43543);
#12560=VERTEX_POINT('',#43547);
#12561=VERTEX_POINT('',#43551);
#12562=VERTEX_POINT('',#43555);
#12563=VERTEX_POINT('',#43559);
#12564=VERTEX_POINT('',#43563);
#12565=VERTEX_POINT('',#43567);
#12566=VERTEX_POINT('',#43617);
#12567=VERTEX_POINT('',#43623);
#12568=VERTEX_POINT('',#43625);
#12569=VERTEX_POINT('',#43644);
#12570=VERTEX_POINT('',#43666);
#12571=VERTEX_POINT('',#43667);
#12572=VERTEX_POINT('',#43704);
#12573=VERTEX_POINT('',#43710);
#12574=VERTEX_POINT('',#43715);
#12575=VERTEX_POINT('',#43722);
#12576=VERTEX_POINT('',#43727);
#12577=VERTEX_POINT('',#43732);
#15523=EDGE_CURVE('',#12425,#12425,#1111,.T.);
#15524=EDGE_CURVE('',#12425,#12426,#7754,.T.);
#15525=EDGE_CURVE('',#12426,#12426,#1112,.T.);
#15526=EDGE_CURVE('',#12427,#12428,#7755,.T.);
#15527=EDGE_CURVE('',#12429,#12427,#7756,.T.);
#15528=EDGE_CURVE('',#12430,#12429,#1113,.T.);
#15529=EDGE_CURVE('',#12431,#12430,#7757,.T.);
#15530=EDGE_CURVE('',#12432,#12431,#1114,.T.);
#15531=EDGE_CURVE('',#12433,#12432,#7758,.T.);
#15532=EDGE_CURVE('',#12434,#12433,#1115,.T.);
#15533=EDGE_CURVE('',#12435,#12434,#7759,.T.);
#15534=EDGE_CURVE('',#12436,#12435,#1116,.T.);
#15535=EDGE_CURVE('',#12437,#12436,#7760,.T.);
#15536=EDGE_CURVE('',#12438,#12437,#1117,.T.);
#15537=EDGE_CURVE('',#12439,#12438,#7761,.T.);
#15538=EDGE_CURVE('',#12440,#12439,#1118,.T.);
#15539=EDGE_CURVE('',#12441,#12440,#7762,.T.);
#15540=EDGE_CURVE('',#12442,#12441,#1119,.T.);
#15541=EDGE_CURVE('',#12443,#12442,#7763,.T.);
#15542=EDGE_CURVE('',#12444,#12443,#1120,.T.);
#15543=EDGE_CURVE('',#12445,#12444,#7764,.T.);
#15544=EDGE_CURVE('',#12446,#12445,#1121,.T.);
#15545=EDGE_CURVE('',#12447,#12446,#7765,.T.);
#15546=EDGE_CURVE('',#12448,#12447,#1122,.T.);
#15547=EDGE_CURVE('',#12449,#12448,#7766,.T.);
#15548=EDGE_CURVE('',#12450,#12449,#1123,.T.);
#15549=EDGE_CURVE('',#12451,#12450,#7767,.T.);
#15550=EDGE_CURVE('',#12428,#12451,#1124,.T.);
#15551=EDGE_CURVE('',#12452,#12452,#1125,.T.);
#15552=EDGE_CURVE('',#12453,#12453,#1126,.T.);
#15553=EDGE_CURVE('',#12454,#12454,#1127,.T.);
#15554=EDGE_CURVE('',#12455,#12455,#1128,.T.);
#15555=EDGE_CURVE('',#12456,#12456,#1129,.T.);
#15556=EDGE_CURVE('',#12457,#12457,#1130,.T.);
#15557=EDGE_CURVE('',#12458,#12458,#1131,.T.);
#15558=EDGE_CURVE('',#12459,#12459,#1132,.T.);
#15559=EDGE_CURVE('',#12460,#12460,#1133,.T.);
#15560=EDGE_CURVE('',#12426,#12461,#7768,.T.);
#15561=EDGE_CURVE('',#12461,#12461,#1134,.T.);
#15562=EDGE_CURVE('',#12452,#12462,#7769,.T.);
#15563=EDGE_CURVE('',#12462,#12462,#1135,.T.);
#15564=EDGE_CURVE('',#12462,#12463,#7770,.T.);
#15565=EDGE_CURVE('',#12463,#12463,#1136,.T.);
#15566=EDGE_CURVE('',#12427,#12464,#7771,.F.);
#15567=EDGE_CURVE('',#12464,#12465,#7772,.T.);
#15568=EDGE_CURVE('',#12465,#12429,#7773,.T.);
#15569=EDGE_CURVE('',#12465,#12466,#1137,.T.);
#15570=EDGE_CURVE('',#12466,#12430,#7774,.T.);
#15571=EDGE_CURVE('',#12467,#12431,#7775,.T.);
#15572=EDGE_CURVE('',#12466,#12467,#7776,.T.);
#15573=EDGE_CURVE('',#12467,#12468,#1138,.T.);
#15574=EDGE_CURVE('',#12468,#12432,#7777,.T.);
#15575=EDGE_CURVE('',#12469,#12433,#162,.T.);
#15576=EDGE_CURVE('',#12468,#12470,#7778,.T.);
#15577=EDGE_CURVE('',#12470,#12469,#7779,.T.);
#15578=EDGE_CURVE('',#12471,#12469,#163,.T.);
#15579=EDGE_CURVE('',#12471,#12472,#1139,.T.);
#15580=EDGE_CURVE('',#12473,#12472,#164,.T.);
#15581=EDGE_CURVE('',#12434,#12473,#2303,.T.);
#15582=EDGE_CURVE('',#12470,#12474,#7780,.T.);
#15583=EDGE_CURVE('',#12474,#12475,#7781,.T.);
#15584=EDGE_CURVE('',#12475,#12471,#7782,.T.);
#15585=EDGE_CURVE('',#12475,#12476,#165,.F.);
#15586=EDGE_CURVE('',#12476,#12474,#7783,.T.);
#15587=EDGE_CURVE('',#12477,#12478,#7784,.F.);
#15588=EDGE_CURVE('',#12478,#12479,#7785,.T.);
#15589=EDGE_CURVE('',#12479,#12480,#7786,.T.);
#15590=EDGE_CURVE('',#12480,#12477,#7787,.T.);
#15591=EDGE_CURVE('',#12481,#12482,#7788,.T.);
#15592=EDGE_CURVE('',#12482,#12480,#1140,.T.);
#15593=EDGE_CURVE('',#12479,#12481,#1141,.T.);
#15594=EDGE_CURVE('',#12483,#12484,#7789,.T.);
#15595=EDGE_CURVE('',#12484,#12482,#7790,.T.);
#15596=EDGE_CURVE('',#12481,#12483,#7791,.T.);
#15597=EDGE_CURVE('',#12485,#12486,#7792,.T.);
#15598=EDGE_CURVE('',#12486,#12484,#1142,.T.);
#15599=EDGE_CURVE('',#12483,#12485,#1143,.T.);
#15600=EDGE_CURVE('',#12485,#12476,#7793,.T.);
#15601=EDGE_CURVE('',#12474,#12486,#7794,.T.);
#15602=EDGE_CURVE('',#12487,#12488,#166,.T.);
#15603=EDGE_CURVE('',#12488,#12475,#1144,.T.);
#15604=EDGE_CURVE('',#12476,#12489,#1145,.T.);
#15605=EDGE_CURVE('',#12489,#12487,#167,.T.);
#15606=EDGE_CURVE('',#12482,#12466,#7795,.T.);
#15607=EDGE_CURVE('',#12467,#12484,#7796,.T.);
#15608=EDGE_CURVE('',#12486,#12468,#7797,.T.);
#15609=EDGE_CURVE('',#12472,#12488,#7798,.T.);
#15610=EDGE_CURVE('',#12490,#12487,#7799,.T.);
#15611=EDGE_CURVE('',#12490,#12491,#7800,.T.);
#15612=EDGE_CURVE('',#12491,#12473,#7801,.T.);
#15613=EDGE_CURVE('',#12489,#12492,#7802,.T.);
#15614=EDGE_CURVE('',#12492,#12493,#7803,.T.);
#15615=EDGE_CURVE('',#12493,#12490,#7804,.T.);
#15616=EDGE_CURVE('',#12494,#12494,#1146,.T.);
#15617=EDGE_CURVE('',#12494,#12495,#7805,.T.);
#15618=EDGE_CURVE('',#12495,#12495,#1147,.T.);
#15619=EDGE_CURVE('',#12478,#12496,#7806,.T.);
#15620=EDGE_CURVE('',#12497,#12496,#1148,.F.);
#15621=EDGE_CURVE('',#12497,#12498,#7807,.T.);
#15622=EDGE_CURVE('',#12499,#12498,#1149,.T.);
#15623=EDGE_CURVE('',#12500,#12499,#7808,.T.);
#15624=EDGE_CURVE('',#12501,#12500,#1150,.T.);
#15625=EDGE_CURVE('',#12502,#12501,#7809,.T.);
#15626=EDGE_CURVE('',#12503,#12502,#1151,.T.);
#15627=EDGE_CURVE('',#12504,#12503,#7810,.T.);
#15628=EDGE_CURVE('',#12505,#12504,#1152,.T.);
#15629=EDGE_CURVE('',#12506,#12505,#7811,.T.);
#15630=EDGE_CURVE('',#12507,#12506,#1153,.T.);
#15631=EDGE_CURVE('',#12508,#12507,#7812,.T.);
#15632=EDGE_CURVE('',#12492,#12508,#1154,.T.);
#15633=EDGE_CURVE('',#12509,#12509,#1155,.T.);
#15634=EDGE_CURVE('',#12510,#12510,#1156,.T.);
#15635=EDGE_CURVE('',#12511,#12511,#1157,.T.);
#15636=EDGE_CURVE('',#12512,#12512,#1158,.T.);
#15637=EDGE_CURVE('',#12512,#12495,#7813,.T.);
#15638=EDGE_CURVE('',#12509,#12513,#7814,.T.);
#15639=EDGE_CURVE('',#12513,#12513,#1159,.T.);
#15640=EDGE_CURVE('',#12514,#12514,#1160,.T.);
#15641=EDGE_CURVE('',#12514,#12513,#7815,.T.);
#15642=EDGE_CURVE('',#12511,#12515,#7816,.T.);
#15643=EDGE_CURVE('',#12515,#12515,#1161,.T.);
#15644=EDGE_CURVE('',#12516,#12516,#1162,.T.);
#15645=EDGE_CURVE('',#12516,#12515,#7817,.T.);
#15646=EDGE_CURVE('',#12508,#12517,#7818,.T.);
#15647=EDGE_CURVE('',#12517,#12493,#1163,.T.);
#15648=EDGE_CURVE('',#12507,#12518,#7819,.T.);
#15649=EDGE_CURVE('',#12518,#12517,#7820,.T.);
#15650=EDGE_CURVE('',#12506,#12519,#7821,.T.);
#15651=EDGE_CURVE('',#12519,#12518,#1164,.T.);
#15652=EDGE_CURVE('',#12505,#12520,#7822,.T.);
#15653=EDGE_CURVE('',#12520,#12519,#7823,.T.);
#15654=EDGE_CURVE('',#12504,#12521,#7824,.T.);
#15655=EDGE_CURVE('',#12521,#12520,#1165,.T.);
#15656=EDGE_CURVE('',#12503,#12522,#7825,.T.);
#15657=EDGE_CURVE('',#12522,#12521,#7826,.T.);
#15658=EDGE_CURVE('',#12502,#12523,#7827,.T.);
#15659=EDGE_CURVE('',#12523,#12522,#1166,.T.);
#15660=EDGE_CURVE('',#12501,#12524,#7828,.T.);
#15661=EDGE_CURVE('',#12524,#12523,#7829,.T.);
#15662=EDGE_CURVE('',#12500,#12525,#7830,.T.);
#15663=EDGE_CURVE('',#12525,#12524,#1167,.T.);
#15664=EDGE_CURVE('',#12499,#12526,#7831,.T.);
#15665=EDGE_CURVE('',#12526,#12525,#7832,.T.);
#15666=EDGE_CURVE('',#12498,#12527,#168,.F.);
#15667=EDGE_CURVE('',#12527,#12526,#1168,.T.);
#15668=EDGE_CURVE('',#12491,#12528,#7833,.T.);
#15669=EDGE_CURVE('',#12528,#12435,#7834,.T.);
#15670=EDGE_CURVE('',#12529,#12530,#7835,.T.);
#15671=EDGE_CURVE('',#12530,#12531,#7836,.T.);
#15672=EDGE_CURVE('',#12531,#12532,#7837,.T.);
#15673=EDGE_CURVE('',#12532,#12529,#7838,.T.);
#15674=EDGE_CURVE('',#12533,#12534,#7839,.T.);
#15675=EDGE_CURVE('',#12534,#12530,#1169,.T.);
#15676=EDGE_CURVE('',#12529,#12533,#1170,.T.);
#15677=EDGE_CURVE('',#12535,#12536,#7840,.T.);
#15678=EDGE_CURVE('',#12536,#12534,#7841,.T.);
#15679=EDGE_CURVE('',#12533,#12535,#7842,.T.);
#15680=EDGE_CURVE('',#12537,#12538,#7843,.T.);
#15681=EDGE_CURVE('',#12538,#12536,#1171,.T.);
#15682=EDGE_CURVE('',#12535,#12537,#1172,.T.);
#15683=EDGE_CURVE('',#12539,#12540,#7844,.T.);
#15684=EDGE_CURVE('',#12540,#12538,#7845,.T.);
#15685=EDGE_CURVE('',#12537,#12539,#7846,.T.);
#15686=EDGE_CURVE('',#12541,#12542,#7847,.T.);
#15687=EDGE_CURVE('',#12542,#12540,#1173,.T.);
#15688=EDGE_CURVE('',#12539,#12541,#1174,.T.);
#15689=EDGE_CURVE('',#12543,#12544,#7848,.T.);
#15690=EDGE_CURVE('',#12544,#12542,#7849,.T.);
#15691=EDGE_CURVE('',#12541,#12543,#7850,.T.);
#15692=EDGE_CURVE('',#12531,#12544,#1175,.T.);
#15693=EDGE_CURVE('',#12543,#12532,#1176,.T.);
#15694=EDGE_CURVE('',#12542,#12545,#7851,.T.);
#15695=EDGE_CURVE('',#12546,#12545,#1177,.T.);
#15696=EDGE_CURVE('',#12546,#12540,#7852,.T.);
#15697=EDGE_CURVE('',#12547,#12544,#7853,.T.);
#15698=EDGE_CURVE('',#12545,#12547,#7854,.T.);
#15699=EDGE_CURVE('',#12531,#12548,#7855,.T.);
#15700=EDGE_CURVE('',#12548,#12549,#2304,.T.);
#15701=EDGE_CURVE('',#12549,#12550,#7856,.T.);
#15702=EDGE_CURVE('',#12547,#12550,#1178,.T.);
#15703=EDGE_CURVE('',#12496,#12530,#7857,.T.);
#15704=EDGE_CURVE('',#12477,#12464,#7858,.T.);
#15705=EDGE_CURVE('',#12550,#12464,#7859,.T.);
#15706=EDGE_CURVE('',#12549,#12551,#1179,.T.);
#15707=EDGE_CURVE('',#12551,#12548,#1180,.T.);
#15708=EDGE_CURVE('',#12552,#12552,#1181,.T.);
#15709=EDGE_CURVE('',#12528,#12553,#1182,.T.);
#15710=EDGE_CURVE('',#12553,#12436,#7860,.T.);
#15711=EDGE_CURVE('',#12554,#12437,#7861,.T.);
#15712=EDGE_CURVE('',#12553,#12554,#7862,.T.);
#15713=EDGE_CURVE('',#12554,#12555,#1183,.T.);
#15714=EDGE_CURVE('',#12555,#12438,#7863,.T.);
#15715=EDGE_CURVE('',#12556,#12439,#7864,.T.);
#15716=EDGE_CURVE('',#12555,#12556,#7865,.T.);
#15717=EDGE_CURVE('',#12556,#12557,#1184,.T.);
#15718=EDGE_CURVE('',#12557,#12440,#7866,.T.);
#15719=EDGE_CURVE('',#12558,#12441,#7867,.T.);
#15720=EDGE_CURVE('',#12557,#12558,#7868,.T.);
#15721=EDGE_CURVE('',#12558,#12559,#1185,.T.);
#15722=EDGE_CURVE('',#12559,#12442,#7869,.T.);
#15723=EDGE_CURVE('',#12560,#12443,#7870,.T.);
#15724=EDGE_CURVE('',#12559,#12560,#7871,.T.);
#15725=EDGE_CURVE('',#12560,#12561,#1186,.T.);
#15726=EDGE_CURVE('',#12561,#12444,#7872,.T.);
#15727=EDGE_CURVE('',#12562,#12445,#7873,.T.);
#15728=EDGE_CURVE('',#12561,#12562,#7874,.T.);
#15729=EDGE_CURVE('',#12562,#12563,#1187,.T.);
#15730=EDGE_CURVE('',#12563,#12446,#7875,.T.);
#15731=EDGE_CURVE('',#12564,#12447,#7876,.T.);
#15732=EDGE_CURVE('',#12563,#12564,#7877,.T.);
#15733=EDGE_CURVE('',#12564,#12565,#1188,.T.);
#15734=EDGE_CURVE('',#12565,#12448,#7878,.T.);
#15735=EDGE_CURVE('',#12546,#12449,#7879,.T.);
#15736=EDGE_CURVE('',#12565,#12546,#7880,.T.);
#15737=EDGE_CURVE('',#12545,#12450,#7881,.T.);
#15738=EDGE_CURVE('',#12547,#12451,#7882,.T.);
#15739=EDGE_CURVE('',#12550,#12428,#7883,.T.);
#15740=EDGE_CURVE('',#12538,#12565,#7884,.T.);
#15741=EDGE_CURVE('',#12564,#12536,#7885,.T.);
#15742=EDGE_CURVE('',#12527,#12563,#7886,.T.);
#15743=EDGE_CURVE('',#12534,#12497,#7887,.T.);
#15744=EDGE_CURVE('',#12562,#12526,#7888,.T.);
#15745=EDGE_CURVE('',#12525,#12561,#7889,.T.);
#15746=EDGE_CURVE('',#12560,#12524,#7890,.T.);
#15747=EDGE_CURVE('',#12523,#12559,#7891,.T.);
#15748=EDGE_CURVE('',#12558,#12522,#7892,.T.);
#15749=EDGE_CURVE('',#12521,#12557,#7893,.T.);
#15750=EDGE_CURVE('',#12556,#12520,#7894,.T.);
#15751=EDGE_CURVE('',#12519,#12555,#7895,.T.);
#15752=EDGE_CURVE('',#12554,#12518,#7896,.T.);
#15753=EDGE_CURVE('',#12517,#12553,#7897,.T.);
#15754=EDGE_CURVE('',#12528,#12493,#7898,.T.);
#15755=EDGE_CURVE('',#12453,#12516,#7899,.T.);
#15756=EDGE_CURVE('',#12460,#12514,#7900,.T.);
#15757=EDGE_CURVE('',#12454,#12512,#7901,.T.);
#15758=EDGE_CURVE('',#12459,#12566,#7902,.T.);
#15759=EDGE_CURVE('',#12566,#12566,#1189,.T.);
#15760=EDGE_CURVE('',#12566,#12510,#7903,.T.);
#15761=EDGE_CURVE('',#12455,#12567,#7904,.T.);
#15762=EDGE_CURVE('',#12568,#12567,#2305,.T.);
#15763=EDGE_CURVE('',#12569,#12568,#2306,.T.);
#15764=EDGE_CURVE('',#12567,#12569,#2307,.T.);
#15765=EDGE_CURVE('',#12570,#12571,#2308,.T.);
#15766=EDGE_CURVE('',#12571,#12570,#2309,.T.);
#15767=EDGE_CURVE('',#12571,#12572,#7905,.T.);
#15768=EDGE_CURVE('',#12572,#12572,#1190,.T.);
#15769=EDGE_CURVE('',#12551,#12568,#7906,.T.);
#15770=EDGE_CURVE('',#12567,#12573,#7907,.T.);
#15771=EDGE_CURVE('',#12573,#12573,#1191,.T.);
#15772=EDGE_CURVE('',#12552,#12574,#7908,.T.);
#15773=EDGE_CURVE('',#12574,#12574,#1192,.T.);
#15774=EDGE_CURVE('',#12458,#12575,#7909,.T.);
#15775=EDGE_CURVE('',#12575,#12575,#1193,.T.);
#15776=EDGE_CURVE('',#12457,#12576,#7910,.T.);
#15777=EDGE_CURVE('',#12576,#12576,#1194,.T.);
#15778=EDGE_CURVE('',#12456,#12577,#7911,.T.);
#15779=EDGE_CURVE('',#12577,#12577,#1195,.T.);
#15780=EDGE_CURVE('',#12465,#12480,#7912,.T.);
#20603=ORIENTED_EDGE('',*,*,#15523,.T.);
#20604=ORIENTED_EDGE('',*,*,#15524,.T.);
#20605=ORIENTED_EDGE('',*,*,#15525,.T.);
#20606=ORIENTED_EDGE('',*,*,#15524,.F.);
#20607=ORIENTED_EDGE('',*,*,#15526,.F.);
#20608=ORIENTED_EDGE('',*,*,#15527,.F.);
#20609=ORIENTED_EDGE('',*,*,#15528,.F.);
#20610=ORIENTED_EDGE('',*,*,#15529,.F.);
#20611=ORIENTED_EDGE('',*,*,#15530,.F.);
#20612=ORIENTED_EDGE('',*,*,#15531,.F.);
#20613=ORIENTED_EDGE('',*,*,#15532,.F.);
#20614=ORIENTED_EDGE('',*,*,#15533,.F.);
#20615=ORIENTED_EDGE('',*,*,#15534,.F.);
#20616=ORIENTED_EDGE('',*,*,#15535,.F.);
#20617=ORIENTED_EDGE('',*,*,#15536,.F.);
#20618=ORIENTED_EDGE('',*,*,#15537,.F.);
#20619=ORIENTED_EDGE('',*,*,#15538,.F.);
#20620=ORIENTED_EDGE('',*,*,#15539,.F.);
#20621=ORIENTED_EDGE('',*,*,#15540,.F.);
#20622=ORIENTED_EDGE('',*,*,#15541,.F.);
#20623=ORIENTED_EDGE('',*,*,#15542,.F.);
#20624=ORIENTED_EDGE('',*,*,#15543,.F.);
#20625=ORIENTED_EDGE('',*,*,#15544,.F.);
#20626=ORIENTED_EDGE('',*,*,#15545,.F.);
#20627=ORIENTED_EDGE('',*,*,#15546,.F.);
#20628=ORIENTED_EDGE('',*,*,#15547,.F.);
#20629=ORIENTED_EDGE('',*,*,#15548,.F.);
#20630=ORIENTED_EDGE('',*,*,#15549,.F.);
#20631=ORIENTED_EDGE('',*,*,#15550,.F.);
#20632=ORIENTED_EDGE('',*,*,#15551,.F.);
#20633=ORIENTED_EDGE('',*,*,#15552,.F.);
#20634=ORIENTED_EDGE('',*,*,#15553,.F.);
#20635=ORIENTED_EDGE('',*,*,#15554,.T.);
#20636=ORIENTED_EDGE('',*,*,#15555,.T.);
#20637=ORIENTED_EDGE('',*,*,#15556,.T.);
#20638=ORIENTED_EDGE('',*,*,#15557,.T.);
#20639=ORIENTED_EDGE('',*,*,#15558,.F.);
#20640=ORIENTED_EDGE('',*,*,#15559,.F.);
#20641=ORIENTED_EDGE('',*,*,#15523,.F.);
#20642=ORIENTED_EDGE('',*,*,#15525,.F.);
#20643=ORIENTED_EDGE('',*,*,#15560,.T.);
#20644=ORIENTED_EDGE('',*,*,#15561,.T.);
#20645=ORIENTED_EDGE('',*,*,#15560,.F.);
#20646=ORIENTED_EDGE('',*,*,#15551,.T.);
#20647=ORIENTED_EDGE('',*,*,#15562,.T.);
#20648=ORIENTED_EDGE('',*,*,#15563,.T.);
#20649=ORIENTED_EDGE('',*,*,#15562,.F.);
#20650=ORIENTED_EDGE('',*,*,#15563,.F.);
#20651=ORIENTED_EDGE('',*,*,#15564,.T.);
#20652=ORIENTED_EDGE('',*,*,#15565,.T.);
#20653=ORIENTED_EDGE('',*,*,#15564,.F.);
#20654=ORIENTED_EDGE('',*,*,#15566,.T.);
#20655=ORIENTED_EDGE('',*,*,#15567,.T.);
#20656=ORIENTED_EDGE('',*,*,#15568,.T.);
#20657=ORIENTED_EDGE('',*,*,#15527,.T.);
#20658=ORIENTED_EDGE('',*,*,#15568,.F.);
#20659=ORIENTED_EDGE('',*,*,#15569,.T.);
#20660=ORIENTED_EDGE('',*,*,#15570,.T.);
#20661=ORIENTED_EDGE('',*,*,#15528,.T.);
#20662=ORIENTED_EDGE('',*,*,#15571,.T.);
#20663=ORIENTED_EDGE('',*,*,#15529,.T.);
#20664=ORIENTED_EDGE('',*,*,#15570,.F.);
#20665=ORIENTED_EDGE('',*,*,#15572,.T.);
#20666=ORIENTED_EDGE('',*,*,#15571,.F.);
#20667=ORIENTED_EDGE('',*,*,#15573,.T.);
#20668=ORIENTED_EDGE('',*,*,#15574,.T.);
#20669=ORIENTED_EDGE('',*,*,#15530,.T.);
#20670=ORIENTED_EDGE('',*,*,#15575,.T.);
#20671=ORIENTED_EDGE('',*,*,#15531,.T.);
#20672=ORIENTED_EDGE('',*,*,#15574,.F.);
#20673=ORIENTED_EDGE('',*,*,#15576,.T.);
#20674=ORIENTED_EDGE('',*,*,#15577,.T.);
#20675=ORIENTED_EDGE('',*,*,#15575,.F.);
#20676=ORIENTED_EDGE('',*,*,#15578,.F.);
#20677=ORIENTED_EDGE('',*,*,#15579,.T.);
#20678=ORIENTED_EDGE('',*,*,#15580,.F.);
#20679=ORIENTED_EDGE('',*,*,#15581,.F.);
#20680=ORIENTED_EDGE('',*,*,#15532,.T.);
#20681=ORIENTED_EDGE('',*,*,#15577,.F.);
#20682=ORIENTED_EDGE('',*,*,#15582,.T.);
#20683=ORIENTED_EDGE('',*,*,#15583,.T.);
#20684=ORIENTED_EDGE('',*,*,#15584,.T.);
#20685=ORIENTED_EDGE('',*,*,#15578,.T.);
#20686=ORIENTED_EDGE('',*,*,#15585,.F.);
#20687=ORIENTED_EDGE('',*,*,#15583,.F.);
#20688=ORIENTED_EDGE('',*,*,#15586,.F.);
#20689=ORIENTED_EDGE('',*,*,#15587,.T.);
#20690=ORIENTED_EDGE('',*,*,#15588,.T.);
#20691=ORIENTED_EDGE('',*,*,#15589,.T.);
#20692=ORIENTED_EDGE('',*,*,#15590,.T.);
#20693=ORIENTED_EDGE('',*,*,#15591,.T.);
#20694=ORIENTED_EDGE('',*,*,#15592,.T.);
#20695=ORIENTED_EDGE('',*,*,#15589,.F.);
#20696=ORIENTED_EDGE('',*,*,#15593,.T.);
#20697=ORIENTED_EDGE('',*,*,#15594,.T.);
#20698=ORIENTED_EDGE('',*,*,#15595,.T.);
#20699=ORIENTED_EDGE('',*,*,#15591,.F.);
#20700=ORIENTED_EDGE('',*,*,#15596,.T.);
#20701=ORIENTED_EDGE('',*,*,#15597,.T.);
#20702=ORIENTED_EDGE('',*,*,#15598,.T.);
#20703=ORIENTED_EDGE('',*,*,#15594,.F.);
#20704=ORIENTED_EDGE('',*,*,#15599,.T.);
#20705=ORIENTED_EDGE('',*,*,#15597,.F.);
#20706=ORIENTED_EDGE('',*,*,#15600,.T.);
#20707=ORIENTED_EDGE('',*,*,#15586,.T.);
#20708=ORIENTED_EDGE('',*,*,#15601,.T.);
#20709=ORIENTED_EDGE('',*,*,#15602,.T.);
#20710=ORIENTED_EDGE('',*,*,#15603,.T.);
#20711=ORIENTED_EDGE('',*,*,#15585,.T.);
#20712=ORIENTED_EDGE('',*,*,#15604,.T.);
#20713=ORIENTED_EDGE('',*,*,#15605,.T.);
#20714=ORIENTED_EDGE('',*,*,#15572,.F.);
#20715=ORIENTED_EDGE('',*,*,#15606,.F.);
#20716=ORIENTED_EDGE('',*,*,#15595,.F.);
#20717=ORIENTED_EDGE('',*,*,#15607,.F.);
#20718=ORIENTED_EDGE('',*,*,#15573,.F.);
#20719=ORIENTED_EDGE('',*,*,#15607,.T.);
#20720=ORIENTED_EDGE('',*,*,#15598,.F.);
#20721=ORIENTED_EDGE('',*,*,#15608,.T.);
#20722=ORIENTED_EDGE('',*,*,#15576,.F.);
#20723=ORIENTED_EDGE('',*,*,#15608,.F.);
#20724=ORIENTED_EDGE('',*,*,#15601,.F.);
#20725=ORIENTED_EDGE('',*,*,#15582,.F.);
#20726=ORIENTED_EDGE('',*,*,#15584,.F.);
#20727=ORIENTED_EDGE('',*,*,#15603,.F.);
#20728=ORIENTED_EDGE('',*,*,#15609,.F.);
#20729=ORIENTED_EDGE('',*,*,#15579,.F.);
#20730=ORIENTED_EDGE('',*,*,#15602,.F.);
#20731=ORIENTED_EDGE('',*,*,#15610,.F.);
#20732=ORIENTED_EDGE('',*,*,#15611,.T.);
#20733=ORIENTED_EDGE('',*,*,#15612,.T.);
#20734=ORIENTED_EDGE('',*,*,#15580,.T.);
#20735=ORIENTED_EDGE('',*,*,#15609,.T.);
#20736=ORIENTED_EDGE('',*,*,#15605,.F.);
#20737=ORIENTED_EDGE('',*,*,#15613,.T.);
#20738=ORIENTED_EDGE('',*,*,#15614,.T.);
#20739=ORIENTED_EDGE('',*,*,#15615,.T.);
#20740=ORIENTED_EDGE('',*,*,#15610,.T.);
#20741=ORIENTED_EDGE('',*,*,#15616,.T.);
#20742=ORIENTED_EDGE('',*,*,#15617,.T.);
#20743=ORIENTED_EDGE('',*,*,#15618,.T.);
#20744=ORIENTED_EDGE('',*,*,#15617,.F.);
#20745=ORIENTED_EDGE('',*,*,#15588,.F.);
#20746=ORIENTED_EDGE('',*,*,#15619,.T.);
#20747=ORIENTED_EDGE('',*,*,#15620,.F.);
#20748=ORIENTED_EDGE('',*,*,#15621,.T.);
#20749=ORIENTED_EDGE('',*,*,#15622,.F.);
#20750=ORIENTED_EDGE('',*,*,#15623,.F.);
#20751=ORIENTED_EDGE('',*,*,#15624,.F.);
#20752=ORIENTED_EDGE('',*,*,#15625,.F.);
#20753=ORIENTED_EDGE('',*,*,#15626,.F.);
#20754=ORIENTED_EDGE('',*,*,#15627,.F.);
#20755=ORIENTED_EDGE('',*,*,#15628,.F.);
#20756=ORIENTED_EDGE('',*,*,#15629,.F.);
#20757=ORIENTED_EDGE('',*,*,#15630,.F.);
#20758=ORIENTED_EDGE('',*,*,#15631,.F.);
#20759=ORIENTED_EDGE('',*,*,#15632,.F.);
#20760=ORIENTED_EDGE('',*,*,#15613,.F.);
#20761=ORIENTED_EDGE('',*,*,#15604,.F.);
#20762=ORIENTED_EDGE('',*,*,#15600,.F.);
#20763=ORIENTED_EDGE('',*,*,#15599,.F.);
#20764=ORIENTED_EDGE('',*,*,#15596,.F.);
#20765=ORIENTED_EDGE('',*,*,#15593,.F.);
#20766=ORIENTED_EDGE('',*,*,#15633,.F.);
#20767=ORIENTED_EDGE('',*,*,#15634,.T.);
#20768=ORIENTED_EDGE('',*,*,#15635,.F.);
#20769=ORIENTED_EDGE('',*,*,#15616,.F.);
#20770=ORIENTED_EDGE('',*,*,#15636,.F.);
#20771=ORIENTED_EDGE('',*,*,#15637,.T.);
#20772=ORIENTED_EDGE('',*,*,#15618,.F.);
#20773=ORIENTED_EDGE('',*,*,#15637,.F.);
#20774=ORIENTED_EDGE('',*,*,#15633,.T.);
#20775=ORIENTED_EDGE('',*,*,#15638,.T.);
#20776=ORIENTED_EDGE('',*,*,#15639,.T.);
#20777=ORIENTED_EDGE('',*,*,#15638,.F.);
#20778=ORIENTED_EDGE('',*,*,#15640,.F.);
#20779=ORIENTED_EDGE('',*,*,#15641,.T.);
#20780=ORIENTED_EDGE('',*,*,#15639,.F.);
#20781=ORIENTED_EDGE('',*,*,#15641,.F.);
#20782=ORIENTED_EDGE('',*,*,#15635,.T.);
#20783=ORIENTED_EDGE('',*,*,#15642,.T.);
#20784=ORIENTED_EDGE('',*,*,#15643,.T.);
#20785=ORIENTED_EDGE('',*,*,#15642,.F.);
#20786=ORIENTED_EDGE('',*,*,#15644,.F.);
#20787=ORIENTED_EDGE('',*,*,#15645,.T.);
#20788=ORIENTED_EDGE('',*,*,#15643,.F.);
#20789=ORIENTED_EDGE('',*,*,#15645,.F.);
#20790=ORIENTED_EDGE('',*,*,#15646,.T.);
#20791=ORIENTED_EDGE('',*,*,#15647,.T.);
#20792=ORIENTED_EDGE('',*,*,#15614,.F.);
#20793=ORIENTED_EDGE('',*,*,#15632,.T.);
#20794=ORIENTED_EDGE('',*,*,#15648,.T.);
#20795=ORIENTED_EDGE('',*,*,#15649,.T.);
#20796=ORIENTED_EDGE('',*,*,#15646,.F.);
#20797=ORIENTED_EDGE('',*,*,#15631,.T.);
#20798=ORIENTED_EDGE('',*,*,#15650,.T.);
#20799=ORIENTED_EDGE('',*,*,#15651,.T.);
#20800=ORIENTED_EDGE('',*,*,#15648,.F.);
#20801=ORIENTED_EDGE('',*,*,#15630,.T.);
#20802=ORIENTED_EDGE('',*,*,#15652,.T.);
#20803=ORIENTED_EDGE('',*,*,#15653,.T.);
#20804=ORIENTED_EDGE('',*,*,#15650,.F.);
#20805=ORIENTED_EDGE('',*,*,#15629,.T.);
#20806=ORIENTED_EDGE('',*,*,#15654,.T.);
#20807=ORIENTED_EDGE('',*,*,#15655,.T.);
#20808=ORIENTED_EDGE('',*,*,#15652,.F.);
#20809=ORIENTED_EDGE('',*,*,#15628,.T.);
#20810=ORIENTED_EDGE('',*,*,#15656,.T.);
#20811=ORIENTED_EDGE('',*,*,#15657,.T.);
#20812=ORIENTED_EDGE('',*,*,#15654,.F.);
#20813=ORIENTED_EDGE('',*,*,#15627,.T.);
#20814=ORIENTED_EDGE('',*,*,#15658,.T.);
#20815=ORIENTED_EDGE('',*,*,#15659,.T.);
#20816=ORIENTED_EDGE('',*,*,#15656,.F.);
#20817=ORIENTED_EDGE('',*,*,#15626,.T.);
#20818=ORIENTED_EDGE('',*,*,#15660,.T.);
#20819=ORIENTED_EDGE('',*,*,#15661,.T.);
#20820=ORIENTED_EDGE('',*,*,#15658,.F.);
#20821=ORIENTED_EDGE('',*,*,#15625,.T.);
#20822=ORIENTED_EDGE('',*,*,#15662,.T.);
#20823=ORIENTED_EDGE('',*,*,#15663,.T.);
#20824=ORIENTED_EDGE('',*,*,#15660,.F.);
#20825=ORIENTED_EDGE('',*,*,#15624,.T.);
#20826=ORIENTED_EDGE('',*,*,#15664,.T.);
#20827=ORIENTED_EDGE('',*,*,#15665,.T.);
#20828=ORIENTED_EDGE('',*,*,#15662,.F.);
#20829=ORIENTED_EDGE('',*,*,#15623,.T.);
#20830=ORIENTED_EDGE('',*,*,#15666,.T.);
#20831=ORIENTED_EDGE('',*,*,#15667,.T.);
#20832=ORIENTED_EDGE('',*,*,#15664,.F.);
#20833=ORIENTED_EDGE('',*,*,#15622,.T.);
#20834=ORIENTED_EDGE('',*,*,#15612,.F.);
#20835=ORIENTED_EDGE('',*,*,#15668,.T.);
#20836=ORIENTED_EDGE('',*,*,#15669,.T.);
#20837=ORIENTED_EDGE('',*,*,#15533,.T.);
#20838=ORIENTED_EDGE('',*,*,#15581,.T.);
#20839=ORIENTED_EDGE('',*,*,#15670,.T.);
#20840=ORIENTED_EDGE('',*,*,#15671,.T.);
#20841=ORIENTED_EDGE('',*,*,#15672,.T.);
#20842=ORIENTED_EDGE('',*,*,#15673,.T.);
#20843=ORIENTED_EDGE('',*,*,#15674,.T.);
#20844=ORIENTED_EDGE('',*,*,#15675,.T.);
#20845=ORIENTED_EDGE('',*,*,#15670,.F.);
#20846=ORIENTED_EDGE('',*,*,#15676,.T.);
#20847=ORIENTED_EDGE('',*,*,#15677,.T.);
#20848=ORIENTED_EDGE('',*,*,#15678,.T.);
#20849=ORIENTED_EDGE('',*,*,#15674,.F.);
#20850=ORIENTED_EDGE('',*,*,#15679,.T.);
#20851=ORIENTED_EDGE('',*,*,#15680,.T.);
#20852=ORIENTED_EDGE('',*,*,#15681,.T.);
#20853=ORIENTED_EDGE('',*,*,#15677,.F.);
#20854=ORIENTED_EDGE('',*,*,#15682,.T.);
#20855=ORIENTED_EDGE('',*,*,#15683,.T.);
#20856=ORIENTED_EDGE('',*,*,#15684,.T.);
#20857=ORIENTED_EDGE('',*,*,#15680,.F.);
#20858=ORIENTED_EDGE('',*,*,#15685,.T.);
#20859=ORIENTED_EDGE('',*,*,#15686,.T.);
#20860=ORIENTED_EDGE('',*,*,#15687,.T.);
#20861=ORIENTED_EDGE('',*,*,#15683,.F.);
#20862=ORIENTED_EDGE('',*,*,#15688,.T.);
#20863=ORIENTED_EDGE('',*,*,#15689,.T.);
#20864=ORIENTED_EDGE('',*,*,#15690,.T.);
#20865=ORIENTED_EDGE('',*,*,#15686,.F.);
#20866=ORIENTED_EDGE('',*,*,#15691,.T.);
#20867=ORIENTED_EDGE('',*,*,#15672,.F.);
#20868=ORIENTED_EDGE('',*,*,#15692,.T.);
#20869=ORIENTED_EDGE('',*,*,#15689,.F.);
#20870=ORIENTED_EDGE('',*,*,#15693,.T.);
#20871=ORIENTED_EDGE('',*,*,#15687,.F.);
#20872=ORIENTED_EDGE('',*,*,#15694,.T.);
#20873=ORIENTED_EDGE('',*,*,#15695,.F.);
#20874=ORIENTED_EDGE('',*,*,#15696,.T.);
#20875=ORIENTED_EDGE('',*,*,#15690,.F.);
#20876=ORIENTED_EDGE('',*,*,#15697,.F.);
#20877=ORIENTED_EDGE('',*,*,#15698,.F.);
#20878=ORIENTED_EDGE('',*,*,#15694,.F.);
#20879=ORIENTED_EDGE('',*,*,#15692,.F.);
#20880=ORIENTED_EDGE('',*,*,#15699,.T.);
#20881=ORIENTED_EDGE('',*,*,#15700,.T.);
#20882=ORIENTED_EDGE('',*,*,#15701,.T.);
#20883=ORIENTED_EDGE('',*,*,#15702,.F.);
#20884=ORIENTED_EDGE('',*,*,#15697,.T.);
#20885=ORIENTED_EDGE('',*,*,#15671,.F.);
#20886=ORIENTED_EDGE('',*,*,#15703,.F.);
#20887=ORIENTED_EDGE('',*,*,#15619,.F.);
#20888=ORIENTED_EDGE('',*,*,#15587,.F.);
#20889=ORIENTED_EDGE('',*,*,#15704,.T.);
#20890=ORIENTED_EDGE('',*,*,#15705,.F.);
#20891=ORIENTED_EDGE('',*,*,#15701,.F.);
#20892=ORIENTED_EDGE('',*,*,#15706,.T.);
#20893=ORIENTED_EDGE('',*,*,#15707,.T.);
#20894=ORIENTED_EDGE('',*,*,#15699,.F.);
#20895=ORIENTED_EDGE('',*,*,#15708,.T.);
#20896=ORIENTED_EDGE('',*,*,#15673,.F.);
#20897=ORIENTED_EDGE('',*,*,#15693,.F.);
#20898=ORIENTED_EDGE('',*,*,#15691,.F.);
#20899=ORIENTED_EDGE('',*,*,#15688,.F.);
#20900=ORIENTED_EDGE('',*,*,#15685,.F.);
#20901=ORIENTED_EDGE('',*,*,#15682,.F.);
#20902=ORIENTED_EDGE('',*,*,#15679,.F.);
#20903=ORIENTED_EDGE('',*,*,#15676,.F.);
#20904=ORIENTED_EDGE('',*,*,#15669,.F.);
#20905=ORIENTED_EDGE('',*,*,#15709,.T.);
#20906=ORIENTED_EDGE('',*,*,#15710,.T.);
#20907=ORIENTED_EDGE('',*,*,#15534,.T.);
#20908=ORIENTED_EDGE('',*,*,#15711,.T.);
#20909=ORIENTED_EDGE('',*,*,#15535,.T.);
#20910=ORIENTED_EDGE('',*,*,#15710,.F.);
#20911=ORIENTED_EDGE('',*,*,#15712,.T.);
#20912=ORIENTED_EDGE('',*,*,#15711,.F.);
#20913=ORIENTED_EDGE('',*,*,#15713,.T.);
#20914=ORIENTED_EDGE('',*,*,#15714,.T.);
#20915=ORIENTED_EDGE('',*,*,#15536,.T.);
#20916=ORIENTED_EDGE('',*,*,#15715,.T.);
#20917=ORIENTED_EDGE('',*,*,#15537,.T.);
#20918=ORIENTED_EDGE('',*,*,#15714,.F.);
#20919=ORIENTED_EDGE('',*,*,#15716,.T.);
#20920=ORIENTED_EDGE('',*,*,#15715,.F.);
#20921=ORIENTED_EDGE('',*,*,#15717,.T.);
#20922=ORIENTED_EDGE('',*,*,#15718,.T.);
#20923=ORIENTED_EDGE('',*,*,#15538,.T.);
#20924=ORIENTED_EDGE('',*,*,#15719,.T.);
#20925=ORIENTED_EDGE('',*,*,#15539,.T.);
#20926=ORIENTED_EDGE('',*,*,#15718,.F.);
#20927=ORIENTED_EDGE('',*,*,#15720,.T.);
#20928=ORIENTED_EDGE('',*,*,#15719,.F.);
#20929=ORIENTED_EDGE('',*,*,#15721,.T.);
#20930=ORIENTED_EDGE('',*,*,#15722,.T.);
#20931=ORIENTED_EDGE('',*,*,#15540,.T.);
#20932=ORIENTED_EDGE('',*,*,#15723,.T.);
#20933=ORIENTED_EDGE('',*,*,#15541,.T.);
#20934=ORIENTED_EDGE('',*,*,#15722,.F.);
#20935=ORIENTED_EDGE('',*,*,#15724,.T.);
#20936=ORIENTED_EDGE('',*,*,#15723,.F.);
#20937=ORIENTED_EDGE('',*,*,#15725,.T.);
#20938=ORIENTED_EDGE('',*,*,#15726,.T.);
#20939=ORIENTED_EDGE('',*,*,#15542,.T.);
#20940=ORIENTED_EDGE('',*,*,#15727,.T.);
#20941=ORIENTED_EDGE('',*,*,#15543,.T.);
#20942=ORIENTED_EDGE('',*,*,#15726,.F.);
#20943=ORIENTED_EDGE('',*,*,#15728,.T.);
#20944=ORIENTED_EDGE('',*,*,#15727,.F.);
#20945=ORIENTED_EDGE('',*,*,#15729,.T.);
#20946=ORIENTED_EDGE('',*,*,#15730,.T.);
#20947=ORIENTED_EDGE('',*,*,#15544,.T.);
#20948=ORIENTED_EDGE('',*,*,#15731,.T.);
#20949=ORIENTED_EDGE('',*,*,#15545,.T.);
#20950=ORIENTED_EDGE('',*,*,#15730,.F.);
#20951=ORIENTED_EDGE('',*,*,#15732,.T.);
#20952=ORIENTED_EDGE('',*,*,#15731,.F.);
#20953=ORIENTED_EDGE('',*,*,#15733,.T.);
#20954=ORIENTED_EDGE('',*,*,#15734,.T.);
#20955=ORIENTED_EDGE('',*,*,#15546,.T.);
#20956=ORIENTED_EDGE('',*,*,#15735,.T.);
#20957=ORIENTED_EDGE('',*,*,#15547,.T.);
#20958=ORIENTED_EDGE('',*,*,#15734,.F.);
#20959=ORIENTED_EDGE('',*,*,#15736,.T.);
#20960=ORIENTED_EDGE('',*,*,#15735,.F.);
#20961=ORIENTED_EDGE('',*,*,#15695,.T.);
#20962=ORIENTED_EDGE('',*,*,#15737,.T.);
#20963=ORIENTED_EDGE('',*,*,#15548,.T.);
#20964=ORIENTED_EDGE('',*,*,#15738,.T.);
#20965=ORIENTED_EDGE('',*,*,#15549,.T.);
#20966=ORIENTED_EDGE('',*,*,#15737,.F.);
#20967=ORIENTED_EDGE('',*,*,#15698,.T.);
#20968=ORIENTED_EDGE('',*,*,#15738,.F.);
#20969=ORIENTED_EDGE('',*,*,#15702,.T.);
#20970=ORIENTED_EDGE('',*,*,#15739,.T.);
#20971=ORIENTED_EDGE('',*,*,#15550,.T.);
#20972=ORIENTED_EDGE('',*,*,#15526,.T.);
#20973=ORIENTED_EDGE('',*,*,#15739,.F.);
#20974=ORIENTED_EDGE('',*,*,#15705,.T.);
#20975=ORIENTED_EDGE('',*,*,#15566,.F.);
#20976=ORIENTED_EDGE('',*,*,#15684,.F.);
#20977=ORIENTED_EDGE('',*,*,#15696,.F.);
#20978=ORIENTED_EDGE('',*,*,#15736,.F.);
#20979=ORIENTED_EDGE('',*,*,#15740,.F.);
#20980=ORIENTED_EDGE('',*,*,#15681,.F.);
#20981=ORIENTED_EDGE('',*,*,#15740,.T.);
#20982=ORIENTED_EDGE('',*,*,#15733,.F.);
#20983=ORIENTED_EDGE('',*,*,#15741,.T.);
#20984=ORIENTED_EDGE('',*,*,#15678,.F.);
#20985=ORIENTED_EDGE('',*,*,#15741,.F.);
#20986=ORIENTED_EDGE('',*,*,#15732,.F.);
#20987=ORIENTED_EDGE('',*,*,#15742,.F.);
#20988=ORIENTED_EDGE('',*,*,#15666,.F.);
#20989=ORIENTED_EDGE('',*,*,#15621,.F.);
#20990=ORIENTED_EDGE('',*,*,#15743,.F.);
#20991=ORIENTED_EDGE('',*,*,#15667,.F.);
#20992=ORIENTED_EDGE('',*,*,#15742,.T.);
#20993=ORIENTED_EDGE('',*,*,#15729,.F.);
#20994=ORIENTED_EDGE('',*,*,#15744,.T.);
#20995=ORIENTED_EDGE('',*,*,#15665,.F.);
#20996=ORIENTED_EDGE('',*,*,#15744,.F.);
#20997=ORIENTED_EDGE('',*,*,#15728,.F.);
#20998=ORIENTED_EDGE('',*,*,#15745,.F.);
#20999=ORIENTED_EDGE('',*,*,#15663,.F.);
#21000=ORIENTED_EDGE('',*,*,#15745,.T.);
#21001=ORIENTED_EDGE('',*,*,#15725,.F.);
#21002=ORIENTED_EDGE('',*,*,#15746,.T.);
#21003=ORIENTED_EDGE('',*,*,#15661,.F.);
#21004=ORIENTED_EDGE('',*,*,#15746,.F.);
#21005=ORIENTED_EDGE('',*,*,#15724,.F.);
#21006=ORIENTED_EDGE('',*,*,#15747,.F.);
#21007=ORIENTED_EDGE('',*,*,#15659,.F.);
#21008=ORIENTED_EDGE('',*,*,#15747,.T.);
#21009=ORIENTED_EDGE('',*,*,#15721,.F.);
#21010=ORIENTED_EDGE('',*,*,#15748,.T.);
#21011=ORIENTED_EDGE('',*,*,#15657,.F.);
#21012=ORIENTED_EDGE('',*,*,#15748,.F.);
#21013=ORIENTED_EDGE('',*,*,#15720,.F.);
#21014=ORIENTED_EDGE('',*,*,#15749,.F.);
#21015=ORIENTED_EDGE('',*,*,#15655,.F.);
#21016=ORIENTED_EDGE('',*,*,#15749,.T.);
#21017=ORIENTED_EDGE('',*,*,#15717,.F.);
#21018=ORIENTED_EDGE('',*,*,#15750,.T.);
#21019=ORIENTED_EDGE('',*,*,#15653,.F.);
#21020=ORIENTED_EDGE('',*,*,#15750,.F.);
#21021=ORIENTED_EDGE('',*,*,#15716,.F.);
#21022=ORIENTED_EDGE('',*,*,#15751,.F.);
#21023=ORIENTED_EDGE('',*,*,#15651,.F.);
#21024=ORIENTED_EDGE('',*,*,#15751,.T.);
#21025=ORIENTED_EDGE('',*,*,#15713,.F.);
#21026=ORIENTED_EDGE('',*,*,#15752,.T.);
#21027=ORIENTED_EDGE('',*,*,#15649,.F.);
#21028=ORIENTED_EDGE('',*,*,#15752,.F.);
#21029=ORIENTED_EDGE('',*,*,#15712,.F.);
#21030=ORIENTED_EDGE('',*,*,#15753,.F.);
#21031=ORIENTED_EDGE('',*,*,#15647,.F.);
#21032=ORIENTED_EDGE('',*,*,#15753,.T.);
#21033=ORIENTED_EDGE('',*,*,#15709,.F.);
#21034=ORIENTED_EDGE('',*,*,#15754,.T.);
#21035=ORIENTED_EDGE('',*,*,#15615,.F.);
#21036=ORIENTED_EDGE('',*,*,#15754,.F.);
#21037=ORIENTED_EDGE('',*,*,#15668,.F.);
#21038=ORIENTED_EDGE('',*,*,#15611,.F.);
#21039=ORIENTED_EDGE('',*,*,#15552,.T.);
#21040=ORIENTED_EDGE('',*,*,#15755,.T.);
#21041=ORIENTED_EDGE('',*,*,#15644,.T.);
#21042=ORIENTED_EDGE('',*,*,#15755,.F.);
#21043=ORIENTED_EDGE('',*,*,#15559,.T.);
#21044=ORIENTED_EDGE('',*,*,#15756,.T.);
#21045=ORIENTED_EDGE('',*,*,#15640,.T.);
#21046=ORIENTED_EDGE('',*,*,#15756,.F.);
#21047=ORIENTED_EDGE('',*,*,#15553,.T.);
#21048=ORIENTED_EDGE('',*,*,#15757,.T.);
#21049=ORIENTED_EDGE('',*,*,#15636,.T.);
#21050=ORIENTED_EDGE('',*,*,#15757,.F.);
#21051=ORIENTED_EDGE('',*,*,#15558,.T.);
#21052=ORIENTED_EDGE('',*,*,#15758,.T.);
#21053=ORIENTED_EDGE('',*,*,#15759,.T.);
#21054=ORIENTED_EDGE('',*,*,#15758,.F.);
#21055=ORIENTED_EDGE('',*,*,#15759,.F.);
#21056=ORIENTED_EDGE('',*,*,#15760,.T.);
#21057=ORIENTED_EDGE('',*,*,#15634,.F.);
#21058=ORIENTED_EDGE('',*,*,#15760,.F.);
#21059=ORIENTED_EDGE('',*,*,#15554,.F.);
#21060=ORIENTED_EDGE('',*,*,#15761,.T.);
#21061=ORIENTED_EDGE('',*,*,#15762,.F.);
#21062=ORIENTED_EDGE('',*,*,#15763,.F.);
#21063=ORIENTED_EDGE('',*,*,#15764,.F.);
#21064=ORIENTED_EDGE('',*,*,#15761,.F.);
#21065=ORIENTED_EDGE('',*,*,#15765,.F.);
#21066=ORIENTED_EDGE('',*,*,#15766,.F.);
#21067=ORIENTED_EDGE('',*,*,#15767,.T.);
#21068=ORIENTED_EDGE('',*,*,#15768,.T.);
#21069=ORIENTED_EDGE('',*,*,#15767,.F.);
#21070=ORIENTED_EDGE('',*,*,#15768,.F.);
#21071=ORIENTED_EDGE('',*,*,#15700,.F.);
#21072=ORIENTED_EDGE('',*,*,#15707,.F.);
#21073=ORIENTED_EDGE('',*,*,#15769,.T.);
#21074=ORIENTED_EDGE('',*,*,#15762,.T.);
#21075=ORIENTED_EDGE('',*,*,#15770,.T.);
#21076=ORIENTED_EDGE('',*,*,#15771,.T.);
#21077=ORIENTED_EDGE('',*,*,#15770,.F.);
#21078=ORIENTED_EDGE('',*,*,#15764,.T.);
#21079=ORIENTED_EDGE('',*,*,#15763,.T.);
#21080=ORIENTED_EDGE('',*,*,#15769,.F.);
#21081=ORIENTED_EDGE('',*,*,#15706,.F.);
#21082=ORIENTED_EDGE('',*,*,#15765,.T.);
#21083=ORIENTED_EDGE('',*,*,#15766,.T.);
#21084=ORIENTED_EDGE('',*,*,#15771,.F.);
#21085=ORIENTED_EDGE('',*,*,#15708,.F.);
#21086=ORIENTED_EDGE('',*,*,#15772,.T.);
#21087=ORIENTED_EDGE('',*,*,#15773,.T.);
#21088=ORIENTED_EDGE('',*,*,#15772,.F.);
#21089=ORIENTED_EDGE('',*,*,#15773,.F.);
#21090=ORIENTED_EDGE('',*,*,#15565,.F.);
#21091=ORIENTED_EDGE('',*,*,#15561,.F.);
#21092=ORIENTED_EDGE('',*,*,#15557,.F.);
#21093=ORIENTED_EDGE('',*,*,#15774,.T.);
#21094=ORIENTED_EDGE('',*,*,#15775,.T.);
#21095=ORIENTED_EDGE('',*,*,#15774,.F.);
#21096=ORIENTED_EDGE('',*,*,#15775,.F.);
#21097=ORIENTED_EDGE('',*,*,#15556,.F.);
#21098=ORIENTED_EDGE('',*,*,#15776,.T.);
#21099=ORIENTED_EDGE('',*,*,#15777,.T.);
#21100=ORIENTED_EDGE('',*,*,#15776,.F.);
#21101=ORIENTED_EDGE('',*,*,#15777,.F.);
#21102=ORIENTED_EDGE('',*,*,#15555,.F.);
#21103=ORIENTED_EDGE('',*,*,#15778,.T.);
#21104=ORIENTED_EDGE('',*,*,#15779,.T.);
#21105=ORIENTED_EDGE('',*,*,#15778,.F.);
#21106=ORIENTED_EDGE('',*,*,#15779,.F.);
#21107=ORIENTED_EDGE('',*,*,#15569,.F.);
#21108=ORIENTED_EDGE('',*,*,#15780,.T.);
#21109=ORIENTED_EDGE('',*,*,#15592,.F.);
#21110=ORIENTED_EDGE('',*,*,#15606,.T.);
#21111=ORIENTED_EDGE('',*,*,#15567,.F.);
#21112=ORIENTED_EDGE('',*,*,#15704,.F.);
#21113=ORIENTED_EDGE('',*,*,#15590,.F.);
#21114=ORIENTED_EDGE('',*,*,#15780,.F.);
#21115=ORIENTED_EDGE('',*,*,#15675,.F.);
#21116=ORIENTED_EDGE('',*,*,#15743,.T.);
#21117=ORIENTED_EDGE('',*,*,#15620,.T.);
#21118=ORIENTED_EDGE('',*,*,#15703,.T.);
#28199=PLANE('',#31126);
#28200=PLANE('',#31154);
#28201=PLANE('',#31157);
#28202=PLANE('',#31160);
#28203=PLANE('',#31163);
#28204=PLANE('',#31164);
#28205=PLANE('',#31165);
#28206=PLANE('',#31169);
#28207=PLANE('',#31173);
#28208=PLANE('',#31177);
#28209=PLANE('',#31179);
#28210=PLANE('',#31181);
#28211=PLANE('',#31182);
#28212=PLANE('',#31186);
#28213=PLANE('',#31209);
#28214=PLANE('',#31212);
#28215=PLANE('',#31215);
#28216=PLANE('',#31218);
#28217=PLANE('',#31221);
#28218=PLANE('',#31224);
#28219=PLANE('',#31225);
#28220=PLANE('',#31229);
#28221=PLANE('',#31233);
#28222=PLANE('',#31237);
#28223=PLANE('',#31243);
#28224=PLANE('',#31246);
#28225=PLANE('',#31250);
#28226=PLANE('',#31253);
#28227=PLANE('',#31256);
#28228=PLANE('',#31259);
#28229=PLANE('',#31262);
#28230=PLANE('',#31265);
#28231=PLANE('',#31268);
#28232=PLANE('',#31271);
#28233=PLANE('',#31273);
#28234=PLANE('',#31275);
#28235=PLANE('',#31276);
#28236=PLANE('',#31278);
#28237=PLANE('',#31280);
#28238=PLANE('',#31282);
#28239=PLANE('',#31284);
#28240=PLANE('',#31286);
#28241=PLANE('',#31288);
#28242=PLANE('',#31290);
#28243=PLANE('',#31300);
#28244=PLANE('',#31303);
#28245=PLANE('',#31306);
#28246=PLANE('',#31307);
#28247=PLANE('',#31308);
#28248=PLANE('',#31311);
#28249=PLANE('',#31314);
#28250=PLANE('',#31317);
#28251=PLANE('',#31319);
#29170=ADVANCED_FACE('',(#3842),#1899,.F.);
#29171=ADVANCED_FACE('',(#3843,#3321,#3322,#3323,#3324,#3325,#3326,#3327,
#3328,#3329,#3330),#28199,.T.);
#29172=ADVANCED_FACE('',(#3844),#457,.F.);
#29173=ADVANCED_FACE('',(#3845),#1900,.F.);
#29174=ADVANCED_FACE('',(#3846),#458,.F.);
#29175=ADVANCED_FACE('',(#3847),#28200,.T.);
#29176=ADVANCED_FACE('',(#3848),#1901,.T.);
#29177=ADVANCED_FACE('',(#3849),#28201,.T.);
#29178=ADVANCED_FACE('',(#3850),#1902,.F.);
#29179=ADVANCED_FACE('',(#3851),#28202,.T.);
#29180=ADVANCED_FACE('',(#3852),#1903,.F.);
#29181=ADVANCED_FACE('',(#3853),#28203,.T.);
#29182=ADVANCED_FACE('',(#3854),#28204,.T.);
#29183=ADVANCED_FACE('',(#3855),#28205,.T.);
#29184=ADVANCED_FACE('',(#3856),#1904,.T.);
#29185=ADVANCED_FACE('',(#3857),#28206,.T.);
#29186=ADVANCED_FACE('',(#3858),#1905,.F.);
#29187=ADVANCED_FACE('',(#3859),#28207,.T.);
#29188=ADVANCED_FACE('',(#3860),#1906,.F.);
#29189=ADVANCED_FACE('',(#3861),#28208,.T.);
#29190=ADVANCED_FACE('',(#3862),#459,.F.);
#29191=ADVANCED_FACE('',(#3863),#28209,.T.);
#29192=ADVANCED_FACE('',(#3864),#460,.F.);
#29193=ADVANCED_FACE('',(#3865),#28210,.T.);
#29194=ADVANCED_FACE('',(#3866),#28211,.T.);
#29195=ADVANCED_FACE('',(#3867),#1907,.F.);
#29196=ADVANCED_FACE('',(#3868,#3331,#3332,#3333,#3334),#28212,.F.);
#29197=ADVANCED_FACE('',(#3869),#461,.F.);
#29198=ADVANCED_FACE('',(#3870),#1908,.F.);
#29199=ADVANCED_FACE('',(#3871),#462,.F.);
#29200=ADVANCED_FACE('',(#3872),#1909,.F.);
#29201=ADVANCED_FACE('',(#3873),#463,.F.);
#29202=ADVANCED_FACE('',(#3874),#1910,.F.);
#29203=ADVANCED_FACE('',(#3875),#28213,.T.);
#29204=ADVANCED_FACE('',(#3876),#1911,.T.);
#29205=ADVANCED_FACE('',(#3877),#28214,.T.);
#29206=ADVANCED_FACE('',(#3878),#1912,.T.);
#29207=ADVANCED_FACE('',(#3879),#28215,.T.);
#29208=ADVANCED_FACE('',(#3880),#1913,.T.);
#29209=ADVANCED_FACE('',(#3881),#28216,.T.);
#29210=ADVANCED_FACE('',(#3882),#1914,.T.);
#29211=ADVANCED_FACE('',(#3883),#28217,.T.);
#29212=ADVANCED_FACE('',(#3884),#1915,.F.);
#29213=ADVANCED_FACE('',(#3885),#28218,.T.);
#29214=ADVANCED_FACE('',(#3886),#28219,.T.);
#29215=ADVANCED_FACE('',(#3887),#1916,.T.);
#29216=ADVANCED_FACE('',(#3888),#28220,.T.);
#29217=ADVANCED_FACE('',(#3889),#1917,.T.);
#29218=ADVANCED_FACE('',(#3890),#28221,.T.);
#29219=ADVANCED_FACE('',(#3891),#1918,.T.);
#29220=ADVANCED_FACE('',(#3892),#28222,.T.);
#29221=ADVANCED_FACE('',(#3893),#1919,.T.);
#29222=ADVANCED_FACE('',(#3894),#464,.T.);
#29223=ADVANCED_FACE('',(#3895),#28223,.T.);
#29224=ADVANCED_FACE('',(#3896),#465,.T.);
#29225=ADVANCED_FACE('',(#3897,#3335),#28224,.T.);
#29226=ADVANCED_FACE('',(#3898),#28225,.F.);
#29227=ADVANCED_FACE('',(#3899),#1920,.F.);
#29228=ADVANCED_FACE('',(#3900),#28226,.T.);
#29229=ADVANCED_FACE('',(#3901),#1921,.T.);
#29230=ADVANCED_FACE('',(#3902),#28227,.T.);
#29231=ADVANCED_FACE('',(#3903),#1922,.T.);
#29232=ADVANCED_FACE('',(#3904),#28228,.T.);
#29233=ADVANCED_FACE('',(#3905),#1923,.T.);
#29234=ADVANCED_FACE('',(#3906),#28229,.T.);
#29235=ADVANCED_FACE('',(#3907),#1924,.T.);
#29236=ADVANCED_FACE('',(#3908),#28230,.T.);
#29237=ADVANCED_FACE('',(#3909),#1925,.F.);
#29238=ADVANCED_FACE('',(#3910),#28231,.T.);
#29239=ADVANCED_FACE('',(#3911),#1926,.T.);
#29240=ADVANCED_FACE('',(#3912),#28232,.T.);
#29241=ADVANCED_FACE('',(#3913),#1927,.T.);
#29242=ADVANCED_FACE('',(#3914),#28233,.T.);
#29243=ADVANCED_FACE('',(#3915),#1928,.T.);
#29244=ADVANCED_FACE('',(#3916),#28234,.T.);
#29245=ADVANCED_FACE('',(#3917),#28235,.T.);
#29246=ADVANCED_FACE('',(#3918),#466,.T.);
#29247=ADVANCED_FACE('',(#3919),#28236,.T.);
#29248=ADVANCED_FACE('',(#3920),#467,.F.);
#29249=ADVANCED_FACE('',(#3921),#28237,.T.);
#29250=ADVANCED_FACE('',(#3922),#468,.T.);
#29251=ADVANCED_FACE('',(#3923),#28238,.T.);
#29252=ADVANCED_FACE('',(#3924),#469,.T.);
#29253=ADVANCED_FACE('',(#3925),#28239,.T.);
#29254=ADVANCED_FACE('',(#3926),#470,.T.);
#29255=ADVANCED_FACE('',(#3927),#28240,.T.);
#29256=ADVANCED_FACE('',(#3928),#471,.T.);
#29257=ADVANCED_FACE('',(#3929),#28241,.T.);
#29258=ADVANCED_FACE('',(#3930),#472,.F.);
#29259=ADVANCED_FACE('',(#3931),#28242,.T.);
#29260=ADVANCED_FACE('',(#3932),#1929,.F.);
#29261=ADVANCED_FACE('',(#3933),#1930,.F.);
#29262=ADVANCED_FACE('',(#3934),#1931,.F.);
#29263=ADVANCED_FACE('',(#3935),#1932,.F.);
#29264=ADVANCED_FACE('',(#3936),#473,.F.);
#29265=ADVANCED_FACE('',(#3937),#474,.F.);
#29266=ADVANCED_FACE('',(#3938),#475,.F.);
#29267=ADVANCED_FACE('',(#3939),#28243,.T.);
#29268=ADVANCED_FACE('',(#3940,#3336),#476,.F.);
#29269=ADVANCED_FACE('',(#3941),#28244,.T.);
#29270=ADVANCED_FACE('',(#3942),#477,.F.);
#29271=ADVANCED_FACE('',(#3943),#28245,.T.);
#29272=ADVANCED_FACE('',(#3944),#28246,.T.);
#29273=ADVANCED_FACE('',(#3945),#28247,.T.);
#29274=ADVANCED_FACE('',(#3946),#478,.F.);
#29275=ADVANCED_FACE('',(#3947),#28248,.T.);
#29276=ADVANCED_FACE('',(#3948),#479,.F.);
#29277=ADVANCED_FACE('',(#3949),#28249,.T.);
#29278=ADVANCED_FACE('',(#3950),#480,.F.);
#29279=ADVANCED_FACE('',(#3951),#28250,.T.);
#29280=ADVANCED_FACE('',(#3952),#481,.T.);
#29281=ADVANCED_FACE('',(#3953),#28251,.T.);
#29282=ADVANCED_FACE('',(#3954),#482,.T.);
#30662=CLOSED_SHELL('',(#29170,#29171,#29172,#29173,#29174,#29175,#29176,
#29177,#29178,#29179,#29180,#29181,#29182,#29183,#29184,#29185,#29186,#29187,
#29188,#29189,#29190,#29191,#29192,#29193,#29194,#29195,#29196,#29197,#29198,
#29199,#29200,#29201,#29202,#29203,#29204,#29205,#29206,#29207,#29208,#29209,
#29210,#29211,#29212,#29213,#29214,#29215,#29216,#29217,#29218,#29219,#29220,
#29221,#29222,#29223,#29224,#29225,#29226,#29227,#29228,#29229,#29230,#29231,
#29232,#29233,#29234,#29235,#29236,#29237,#29238,#29239,#29240,#29241,#29242,
#29243,#29244,#29245,#29246,#29247,#29248,#29249,#29250,#29251,#29252,#29253,
#29254,#29255,#29256,#29257,#29258,#29259,#29260,#29261,#29262,#29263,#29264,
#29265,#29266,#29267,#29268,#29269,#29270,#29271,#29272,#29273,#29274,#29275,
#29276,#29277,#29278,#29279,#29280,#29281,#29282));
#31122=AXIS2_PLACEMENT_3D('',#43120,#34249,#34250);
#31123=AXIS2_PLACEMENT_3D('',#43121,#34251,#34252);
#31124=AXIS2_PLACEMENT_3D('',#43123,#34253,#34254);
#31125=AXIS2_PLACEMENT_3D('',#43126,#34256,#34257);
#31126=AXIS2_PLACEMENT_3D('',#43127,#34258,#34259);
#31127=AXIS2_PLACEMENT_3D('',#43134,#34262,#34263);
#31128=AXIS2_PLACEMENT_3D('',#43138,#34265,#34266);
#31129=AXIS2_PLACEMENT_3D('',#43142,#34268,#34269);
#31130=AXIS2_PLACEMENT_3D('',#43146,#34271,#34272);
#31131=AXIS2_PLACEMENT_3D('',#43150,#34274,#34275);
#31132=AXIS2_PLACEMENT_3D('',#43154,#34277,#34278);
#31133=AXIS2_PLACEMENT_3D('',#43158,#34280,#34281);
#31134=AXIS2_PLACEMENT_3D('',#43162,#34283,#34284);
#31135=AXIS2_PLACEMENT_3D('',#43166,#34286,#34287);
#31136=AXIS2_PLACEMENT_3D('',#43170,#34289,#34290);
#31137=AXIS2_PLACEMENT_3D('',#43174,#34292,#34293);
#31138=AXIS2_PLACEMENT_3D('',#43177,#34295,#34296);
#31139=AXIS2_PLACEMENT_3D('',#43179,#34297,#34298);
#31140=AXIS2_PLACEMENT_3D('',#43181,#34299,#34300);
#31141=AXIS2_PLACEMENT_3D('',#43183,#34301,#34302);
#31142=AXIS2_PLACEMENT_3D('',#43185,#34303,#34304);
#31143=AXIS2_PLACEMENT_3D('',#43187,#34305,#34306);
#31144=AXIS2_PLACEMENT_3D('',#43189,#34307,#34308);
#31145=AXIS2_PLACEMENT_3D('',#43191,#34309,#34310);
#31146=AXIS2_PLACEMENT_3D('',#43193,#34311,#34312);
#31147=AXIS2_PLACEMENT_3D('',#43195,#34313,#34314);
#31148=AXIS2_PLACEMENT_3D('',#43196,#34315,#34316);
#31149=AXIS2_PLACEMENT_3D('',#43199,#34318,#34319);
#31150=AXIS2_PLACEMENT_3D('',#43200,#34320,#34321);
#31151=AXIS2_PLACEMENT_3D('',#43203,#34323,#34324);
#31152=AXIS2_PLACEMENT_3D('',#43204,#34325,#34326);
#31153=AXIS2_PLACEMENT_3D('',#43207,#34328,#34329);
#31154=AXIS2_PLACEMENT_3D('',#43208,#34330,#34331);
#31155=AXIS2_PLACEMENT_3D('',#43214,#34335,#34336);
#31156=AXIS2_PLACEMENT_3D('',#43216,#34337,#34338);
#31157=AXIS2_PLACEMENT_3D('',#43218,#34340,#34341);
#31158=AXIS2_PLACEMENT_3D('',#43222,#34344,#34345);
#31159=AXIS2_PLACEMENT_3D('',#43224,#34346,#34347);
#31160=AXIS2_PLACEMENT_3D('',#43226,#34349,#34350);
#31161=AXIS2_PLACEMENT_3D('',#43234,#34353,#34354);
#31162=AXIS2_PLACEMENT_3D('',#43240,#34355,#34356);
#31163=AXIS2_PLACEMENT_3D('',#43249,#34357,#34358);
#31164=AXIS2_PLACEMENT_3D('',#43255,#34362,#34363);
#31165=AXIS2_PLACEMENT_3D('',#43261,#34365,#34366);
#31166=AXIS2_PLACEMENT_3D('',#43270,#34371,#34372);
#31167=AXIS2_PLACEMENT_3D('',#43274,#34374,#34375);
#31168=AXIS2_PLACEMENT_3D('',#43275,#34376,#34377);
#31169=AXIS2_PLACEMENT_3D('',#43276,#34378,#34379);
#31170=AXIS2_PLACEMENT_3D('',#43282,#34383,#34384);
#31171=AXIS2_PLACEMENT_3D('',#43286,#34386,#34387);
#31172=AXIS2_PLACEMENT_3D('',#43287,#34388,#34389);
#31173=AXIS2_PLACEMENT_3D('',#43288,#34390,#34391);
#31174=AXIS2_PLACEMENT_3D('',#43291,#34394,#34395);
#31175=AXIS2_PLACEMENT_3D('',#43297,#34396,#34397);
#31176=AXIS2_PLACEMENT_3D('',#43299,#34398,#34399);
#31177=AXIS2_PLACEMENT_3D('',#43303,#34400,#34401);
#31178=AXIS2_PLACEMENT_3D('',#43306,#34404,#34405);
#31179=AXIS2_PLACEMENT_3D('',#43308,#34407,#34408);
#31180=AXIS2_PLACEMENT_3D('',#43309,#34409,#34410);
#31181=AXIS2_PLACEMENT_3D('',#43311,#34412,#34413);
#31182=AXIS2_PLACEMENT_3D('',#43317,#34417,#34418);
#31183=AXIS2_PLACEMENT_3D('',#43323,#34422,#34423);
#31184=AXIS2_PLACEMENT_3D('',#43325,#34424,#34425);
#31185=AXIS2_PLACEMENT_3D('',#43328,#34427,#34428);
#31186=AXIS2_PLACEMENT_3D('',#43329,#34429,#34430);
#31187=AXIS2_PLACEMENT_3D('',#43333,#34432,#34433);
#31188=AXIS2_PLACEMENT_3D('',#43337,#34435,#34436);
#31189=AXIS2_PLACEMENT_3D('',#43341,#34438,#34439);
#31190=AXIS2_PLACEMENT_3D('',#43345,#34441,#34442);
#31191=AXIS2_PLACEMENT_3D('',#43349,#34444,#34445);
#31192=AXIS2_PLACEMENT_3D('',#43353,#34447,#34448);
#31193=AXIS2_PLACEMENT_3D('',#43356,#34450,#34451);
#31194=AXIS2_PLACEMENT_3D('',#43358,#34452,#34453);
#31195=AXIS2_PLACEMENT_3D('',#43360,#34454,#34455);
#31196=AXIS2_PLACEMENT_3D('',#43362,#34456,#34457);
#31197=AXIS2_PLACEMENT_3D('',#43363,#34458,#34459);
#31198=AXIS2_PLACEMENT_3D('',#43365,#34460,#34461);
#31199=AXIS2_PLACEMENT_3D('',#43367,#34463,#34464);
#31200=AXIS2_PLACEMENT_3D('',#43370,#34466,#34467);
#31201=AXIS2_PLACEMENT_3D('',#43371,#34468,#34469);
#31202=AXIS2_PLACEMENT_3D('',#43373,#34470,#34471);
#31203=AXIS2_PLACEMENT_3D('',#43375,#34473,#34474);
#31204=AXIS2_PLACEMENT_3D('',#43378,#34476,#34477);
#31205=AXIS2_PLACEMENT_3D('',#43379,#34478,#34479);
#31206=AXIS2_PLACEMENT_3D('',#43381,#34480,#34481);
#31207=AXIS2_PLACEMENT_3D('',#43383,#34483,#34484);
#31208=AXIS2_PLACEMENT_3D('',#43386,#34486,#34487);
#31209=AXIS2_PLACEMENT_3D('',#43387,#34488,#34489);
#31210=AXIS2_PLACEMENT_3D('',#43391,#34492,#34493);
#31211=AXIS2_PLACEMENT_3D('',#43394,#34495,#34496);
#31212=AXIS2_PLACEMENT_3D('',#43395,#34497,#34498);
#31213=AXIS2_PLACEMENT_3D('',#43399,#34501,#34502);
#31214=AXIS2_PLACEMENT_3D('',#43402,#34504,#34505);
#31215=AXIS2_PLACEMENT_3D('',#43403,#34506,#34507);
#31216=AXIS2_PLACEMENT_3D('',#43407,#34510,#34511);
#31217=AXIS2_PLACEMENT_3D('',#43410,#34513,#34514);
#31218=AXIS2_PLACEMENT_3D('',#43411,#34515,#34516);
#31219=AXIS2_PLACEMENT_3D('',#43415,#34519,#34520);
#31220=AXIS2_PLACEMENT_3D('',#43418,#34522,#34523);
#31221=AXIS2_PLACEMENT_3D('',#43419,#34524,#34525);
#31222=AXIS2_PLACEMENT_3D('',#43423,#34528,#34529);
#31223=AXIS2_PLACEMENT_3D('',#43428,#34530,#34531);
#31224=AXIS2_PLACEMENT_3D('',#43429,#34532,#34533);
#31225=AXIS2_PLACEMENT_3D('',#43433,#34536,#34537);
#31226=AXIS2_PLACEMENT_3D('',#43442,#34542,#34543);
#31227=AXIS2_PLACEMENT_3D('',#43446,#34545,#34546);
#31228=AXIS2_PLACEMENT_3D('',#43447,#34547,#34548);
#31229=AXIS2_PLACEMENT_3D('',#43448,#34549,#34550);
#31230=AXIS2_PLACEMENT_3D('',#43454,#34554,#34555);
#31231=AXIS2_PLACEMENT_3D('',#43458,#34557,#34558);
#31232=AXIS2_PLACEMENT_3D('',#43459,#34559,#34560);
#31233=AXIS2_PLACEMENT_3D('',#43460,#34561,#34562);
#31234=AXIS2_PLACEMENT_3D('',#43466,#34566,#34567);
#31235=AXIS2_PLACEMENT_3D('',#43470,#34569,#34570);
#31236=AXIS2_PLACEMENT_3D('',#43471,#34571,#34572);
#31237=AXIS2_PLACEMENT_3D('',#43472,#34573,#34574);
#31238=AXIS2_PLACEMENT_3D('',#43478,#34578,#34579);
#31239=AXIS2_PLACEMENT_3D('',#43479,#34580,#34581);
#31240=AXIS2_PLACEMENT_3D('',#43480,#34582,#34583);
#31241=AXIS2_PLACEMENT_3D('',#43481,#34584,#34585);
#31242=AXIS2_PLACEMENT_3D('',#43485,#34587,#34588);
#31243=AXIS2_PLACEMENT_3D('',#43487,#34590,#34591);
#31244=AXIS2_PLACEMENT_3D('',#43491,#34594,#34595);
#31245=AXIS2_PLACEMENT_3D('',#43507,#34598,#34599);
#31246=AXIS2_PLACEMENT_3D('',#43508,#34600,#34601);
#31247=AXIS2_PLACEMENT_3D('',#43513,#34605,#34606);
#31248=AXIS2_PLACEMENT_3D('',#43514,#34607,#34608);
#31249=AXIS2_PLACEMENT_3D('',#43516,#34609,#34610);
#31250=AXIS2_PLACEMENT_3D('',#43517,#34611,#34612);
#31251=AXIS2_PLACEMENT_3D('',#43518,#34613,#34614);
#31252=AXIS2_PLACEMENT_3D('',#43520,#34615,#34616);
#31253=AXIS2_PLACEMENT_3D('',#43522,#34618,#34619);
#31254=AXIS2_PLACEMENT_3D('',#43526,#34622,#34623);
#31255=AXIS2_PLACEMENT_3D('',#43528,#34624,#34625);
#31256=AXIS2_PLACEMENT_3D('',#43530,#34627,#34628);
#31257=AXIS2_PLACEMENT_3D('',#43534,#34631,#34632);
#31258=AXIS2_PLACEMENT_3D('',#43536,#34633,#34634);
#31259=AXIS2_PLACEMENT_3D('',#43538,#34636,#34637);
#31260=AXIS2_PLACEMENT_3D('',#43542,#34640,#34641);
#31261=AXIS2_PLACEMENT_3D('',#43544,#34642,#34643);
#31262=AXIS2_PLACEMENT_3D('',#43546,#34645,#34646);
#31263=AXIS2_PLACEMENT_3D('',#43550,#34649,#34650);
#31264=AXIS2_PLACEMENT_3D('',#43552,#34651,#34652);
#31265=AXIS2_PLACEMENT_3D('',#43554,#34654,#34655);
#31266=AXIS2_PLACEMENT_3D('',#43558,#34658,#34659);
#31267=AXIS2_PLACEMENT_3D('',#43560,#34660,#34661);
#31268=AXIS2_PLACEMENT_3D('',#43562,#34663,#34664);
#31269=AXIS2_PLACEMENT_3D('',#43566,#34667,#34668);
#31270=AXIS2_PLACEMENT_3D('',#43568,#34669,#34670);
#31271=AXIS2_PLACEMENT_3D('',#43570,#34672,#34673);
#31272=AXIS2_PLACEMENT_3D('',#43573,#34676,#34677);
#31273=AXIS2_PLACEMENT_3D('',#43575,#34679,#34680);
#31274=AXIS2_PLACEMENT_3D('',#43577,#34682,#34683);
#31275=AXIS2_PLACEMENT_3D('',#43579,#34685,#34686);
#31276=AXIS2_PLACEMENT_3D('',#43580,#34687,#34688);
#31277=AXIS2_PLACEMENT_3D('',#43582,#34690,#34691);
#31278=AXIS2_PLACEMENT_3D('',#43584,#34693,#34694);
#31279=AXIS2_PLACEMENT_3D('',#43587,#34697,#34698);
#31280=AXIS2_PLACEMENT_3D('',#43589,#34700,#34701);
#31281=AXIS2_PLACEMENT_3D('',#43591,#34703,#34704);
#31282=AXIS2_PLACEMENT_3D('',#43593,#34706,#34707);
#31283=AXIS2_PLACEMENT_3D('',#43595,#34709,#34710);
#31284=AXIS2_PLACEMENT_3D('',#43597,#34712,#34713);
#31285=AXIS2_PLACEMENT_3D('',#43599,#34715,#34716);
#31286=AXIS2_PLACEMENT_3D('',#43601,#34718,#34719);
#31287=AXIS2_PLACEMENT_3D('',#43603,#34721,#34722);
#31288=AXIS2_PLACEMENT_3D('',#43605,#34724,#34725);
#31289=AXIS2_PLACEMENT_3D('',#43607,#34727,#34728);
#31290=AXIS2_PLACEMENT_3D('',#43609,#34730,#34731);
#31291=AXIS2_PLACEMENT_3D('',#43610,#34732,#34733);
#31292=AXIS2_PLACEMENT_3D('',#43612,#34735,#34736);
#31293=AXIS2_PLACEMENT_3D('',#43614,#34738,#34739);
#31294=AXIS2_PLACEMENT_3D('',#43616,#34741,#34742);
#31295=AXIS2_PLACEMENT_3D('',#43619,#34744,#34745);
#31296=AXIS2_PLACEMENT_3D('',#43620,#34746,#34747);
#31297=AXIS2_PLACEMENT_3D('',#43622,#34749,#34750);
#31298=AXIS2_PLACEMENT_3D('',#43665,#34752,#34753);
#31299=AXIS2_PLACEMENT_3D('',#43706,#34755,#34756);
#31300=AXIS2_PLACEMENT_3D('',#43707,#34757,#34758);
#31301=AXIS2_PLACEMENT_3D('',#43708,#34759,#34760);
#31302=AXIS2_PLACEMENT_3D('',#43712,#34763,#34764);
#31303=AXIS2_PLACEMENT_3D('',#43713,#34765,#34766);
#31304=AXIS2_PLACEMENT_3D('',#43714,#34767,#34768);
#31305=AXIS2_PLACEMENT_3D('',#43717,#34770,#34771);
#31306=AXIS2_PLACEMENT_3D('',#43718,#34772,#34773);
#31307=AXIS2_PLACEMENT_3D('',#43719,#34774,#34775);
#31308=AXIS2_PLACEMENT_3D('',#43720,#34776,#34777);
#31309=AXIS2_PLACEMENT_3D('',#43721,#34778,#34779);
#31310=AXIS2_PLACEMENT_3D('',#43724,#34781,#34782);
#31311=AXIS2_PLACEMENT_3D('',#43725,#34783,#34784);
#31312=AXIS2_PLACEMENT_3D('',#43726,#34785,#34786);
#31313=AXIS2_PLACEMENT_3D('',#43729,#34788,#34789);
#31314=AXIS2_PLACEMENT_3D('',#43730,#34790,#34791);
#31315=AXIS2_PLACEMENT_3D('',#43731,#34792,#34793);
#31316=AXIS2_PLACEMENT_3D('',#43734,#34795,#34796);
#31317=AXIS2_PLACEMENT_3D('',#43735,#34797,#34798);
#31318=AXIS2_PLACEMENT_3D('',#43736,#34799,#34800);
#31319=AXIS2_PLACEMENT_3D('',#43738,#34802,#34803);
#31320=AXIS2_PLACEMENT_3D('',#43739,#34804,#34805);
#34249=DIRECTION('axis',(0.,0.,1.));
#34250=DIRECTION('refdir',(1.,0.,0.));
#34251=DIRECTION('center_axis',(0.,0.,1.));
#34252=DIRECTION('ref_axis',(1.,0.,0.));
#34253=DIRECTION('center_axis',(0.,0.,1.));
#34254=DIRECTION('ref_axis',(1.,0.,0.));
#34255=DIRECTION('',(0.707106781186547,8.65956056235493E-17,-0.707106781186547));
#34256=DIRECTION('center_axis',(0.,0.,-1.));
#34257=DIRECTION('ref_axis',(1.,0.,0.));
#34258=DIRECTION('center_axis',(0.,0.,1.));
#34259=DIRECTION('ref_axis',(1.,0.,0.));
#34260=DIRECTION('',(0.,-1.,0.));
#34261=DIRECTION('',(-1.,0.,0.));
#34262=DIRECTION('center_axis',(0.,0.,-1.));
#34263=DIRECTION('ref_axis',(0.707106781186545,-0.70710678118655,0.));
#34264=DIRECTION('',(0.,-1.,0.));
#34265=DIRECTION('center_axis',(0.,0.,1.));
#34266=DIRECTION('ref_axis',(-0.70710678118655,0.707106781186545,0.));
#34267=DIRECTION('',(-1.,0.,0.));
#34268=DIRECTION('center_axis',(0.,0.,1.));
#34269=DIRECTION('ref_axis',(1.,0.,0.));
#34270=DIRECTION('',(-1.,0.,0.));
#34271=DIRECTION('center_axis',(0.,0.,1.));
#34272=DIRECTION('ref_axis',(0.707106781186547,0.707106781186547,0.));
#34273=DIRECTION('',(0.,1.,0.));
#34274=DIRECTION('center_axis',(0.,0.,-1.));
#34275=DIRECTION('ref_axis',(-0.70710678118655,-0.707106781186545,0.));
#34276=DIRECTION('',(-1.,0.,0.));
#34277=DIRECTION('center_axis',(0.,0.,-1.));
#34278=DIRECTION('ref_axis',(0.707106781186545,-0.70710678118655,0.));
#34279=DIRECTION('',(0.,-1.,0.));
#34280=DIRECTION('center_axis',(0.,0.,-1.));
#34281=DIRECTION('ref_axis',(0.707106781186548,0.707106781186548,0.));
#34282=DIRECTION('',(1.,0.,0.));
#34283=DIRECTION('center_axis',(0.,0.,-1.));
#34284=DIRECTION('ref_axis',(-0.707106781186548,0.707106781186548,0.));
#34285=DIRECTION('',(0.,1.,0.));
#34286=DIRECTION('center_axis',(0.,0.,1.));
#34287=DIRECTION('ref_axis',(0.707106781186547,-0.707106781186547,0.));
#34288=DIRECTION('',(1.,0.,0.));
#34289=DIRECTION('center_axis',(0.,0.,-1.));
#34290=DIRECTION('ref_axis',(-0.707106781186548,0.707106781186548,0.));
#34291=DIRECTION('',(0.,1.,0.));
#34292=DIRECTION('center_axis',(0.,0.,-1.));
#34293=DIRECTION('ref_axis',(-0.707106781186548,-0.707106781186548,0.));
#34294=DIRECTION('',(-1.,0.,0.));
#34295=DIRECTION('center_axis',(0.,0.,-1.));
#34296=DIRECTION('ref_axis',(0.707106781186545,-0.70710678118655,0.));
#34297=DIRECTION('center_axis',(0.,0.,1.));
#34298=DIRECTION('ref_axis',(1.,0.,0.));
#34299=DIRECTION('center_axis',(0.,0.,1.));
#34300=DIRECTION('ref_axis',(1.,0.,0.));
#34301=DIRECTION('center_axis',(0.,0.,1.));
#34302=DIRECTION('ref_axis',(1.,0.,0.));
#34303=DIRECTION('center_axis',(0.,0.,-1.));
#34304=DIRECTION('ref_axis',(1.,0.,0.));
#34305=DIRECTION('center_axis',(0.,0.,-1.));
#34306=DIRECTION('ref_axis',(1.,0.,0.));
#34307=DIRECTION('center_axis',(0.,0.,-1.));
#34308=DIRECTION('ref_axis',(1.,0.,0.));
#34309=DIRECTION('center_axis',(0.,0.,-1.));
#34310=DIRECTION('ref_axis',(1.,0.,0.));
#34311=DIRECTION('center_axis',(0.,0.,1.));
#34312=DIRECTION('ref_axis',(1.,0.,0.));
#34313=DIRECTION('center_axis',(0.,0.,1.));
#34314=DIRECTION('ref_axis',(1.,0.,0.));
#34315=DIRECTION('center_axis',(0.,0.,-1.));
#34316=DIRECTION('ref_axis',(1.,0.,0.));
#34317=DIRECTION('',(0.,0.,-1.));
#34318=DIRECTION('center_axis',(0.,0.,-1.));
#34319=DIRECTION('ref_axis',(1.,0.,0.));
#34320=DIRECTION('center_axis',(0.,0.,1.));
#34321=DIRECTION('ref_axis',(1.,0.,0.));
#34322=DIRECTION('',(0.707106781186549,8.65956056235495E-17,-0.707106781186546));
#34323=DIRECTION('center_axis',(0.,0.,-1.));
#34324=DIRECTION('ref_axis',(1.,0.,0.));
#34325=DIRECTION('center_axis',(0.,0.,-1.));
#34326=DIRECTION('ref_axis',(1.,0.,0.));
#34327=DIRECTION('',(0.,0.,-1.));
#34328=DIRECTION('center_axis',(0.,0.,-1.));
#34329=DIRECTION('ref_axis',(1.,0.,0.));
#34330=DIRECTION('center_axis',(0.,-0.707106781186548,0.707106781186548));
#34331=DIRECTION('ref_axis',(1.,0.,0.));
#34332=DIRECTION('',(-0.577350269189626,0.577350269189626,0.577350269189626));
#34333=DIRECTION('',(1.,0.,0.));
#34334=DIRECTION('',(0.,0.707106781186548,0.707106781186548));
#34335=DIRECTION('center_axis',(0.,0.,-1.));
#34336=DIRECTION('ref_axis',(0.707106781186545,-0.70710678118655,0.));
#34337=DIRECTION('center_axis',(0.,0.,1.));
#34338=DIRECTION('ref_axis',(0.707106781186545,-0.70710678118655,0.));
#34339=DIRECTION('',(-0.707106781186548,0.,0.707106781186548));
#34340=DIRECTION('center_axis',(0.707106781186548,0.,0.707106781186548));
#34341=DIRECTION('ref_axis',(0.707106781186548,0.,-0.707106781186548));
#34342=DIRECTION('',(-0.707106781186548,0.,0.707106781186548));
#34343=DIRECTION('',(0.,1.,0.));
#34344=DIRECTION('center_axis',(0.,0.,1.));
#34345=DIRECTION('ref_axis',(-0.70710678118655,0.707106781186545,0.));
#34346=DIRECTION('center_axis',(0.,0.,-1.));
#34347=DIRECTION('ref_axis',(-0.70710678118655,0.707106781186545,0.));
#34348=DIRECTION('',(0.,0.707106781186551,0.707106781186544));
#34349=DIRECTION('center_axis',(0.,-0.707106781186548,0.707106781186548));
#34350=DIRECTION('ref_axis',(1.,0.,0.));
#34351=DIRECTION('',(1.,0.,0.));
#34352=DIRECTION('',(0.504717559062642,0.610434347646759,0.610434347646759));
#34353=DIRECTION('center_axis',(0.,0.,1.));
#34354=DIRECTION('ref_axis',(-5.1924747385868E-12,1.,0.));
#34355=DIRECTION('center_axis',(0.,0.,-1.));
#34356=DIRECTION('ref_axis',(1.,0.,0.));
#34357=DIRECTION('center_axis',(0.770685380459105,-0.637215853809841,0.));
#34358=DIRECTION('ref_axis',(0.,0.,-1.));
#34359=DIRECTION('',(0.,0.,-1.));
#34360=DIRECTION('',(0.637215853809841,0.770685380459105,6.96921156614208E-15));
#34361=DIRECTION('',(0.,0.,1.));
#34362=DIRECTION('center_axis',(0.603317169232353,-0.498832954222525,-0.622233137249286));
#34363=DIRECTION('ref_axis',(-0.717935231561239,0.,-0.696109907473748));
#34364=DIRECTION('',(0.143139597747746,-0.699825355198214,0.699825355198214));
#34365=DIRECTION('center_axis',(0.,-0.707106781186548,-0.707106781186548));
#34366=DIRECTION('ref_axis',(-1.,0.,0.));
#34367=DIRECTION('',(0.,-0.707106781186548,0.707106781186548));
#34368=DIRECTION('',(1.,0.,0.));
#34369=DIRECTION('',(0.,-0.707106781186548,0.707106781186548));
#34370=DIRECTION('',(-1.,0.,0.));
#34371=DIRECTION('center_axis',(0.,0.,1.));
#34372=DIRECTION('ref_axis',(0.707106781186545,-0.70710678118655,0.));
#34373=DIRECTION('',(0.707106781186548,0.,0.707106781186548));
#34374=DIRECTION('center_axis',(0.,0.,-1.));
#34375=DIRECTION('ref_axis',(0.707106781186545,-0.70710678118655,0.));
#34376=DIRECTION('center_axis',(0.,0.,1.));
#34377=DIRECTION('ref_axis',(0.707106781186545,-0.70710678118655,0.));
#34378=DIRECTION('center_axis',(0.707106781186548,0.,-0.707106781186548));
#34379=DIRECTION('ref_axis',(-0.707106781186548,0.,-0.707106781186548));
#34380=DIRECTION('',(0.707106781186548,0.,0.707106781186548));
#34381=DIRECTION('',(0.,-1.,0.));
#34382=DIRECTION('',(0.,1.,0.));
#34383=DIRECTION('center_axis',(0.,0.,-1.));
#34384=DIRECTION('ref_axis',(-0.70710678118655,0.707106781186545,0.));
#34385=DIRECTION('',(0.,-0.707106781186551,0.707106781186544));
#34386=DIRECTION('center_axis',(0.,0.,1.));
#34387=DIRECTION('ref_axis',(-0.70710678118655,0.707106781186545,0.));
#34388=DIRECTION('center_axis',(0.,0.,-1.));
#34389=DIRECTION('ref_axis',(-0.70710678118655,0.707106781186545,0.));
#34390=DIRECTION('center_axis',(0.,-0.707106781186548,-0.707106781186548));
#34391=DIRECTION('ref_axis',(-1.,0.,0.));
#34392=DIRECTION('',(1.,0.,0.));
#34393=DIRECTION('',(-1.,0.,0.));
#34394=DIRECTION('center_axis',(0.,0.,-1.));
#34395=DIRECTION('ref_axis',(0.00854146177382261,0.999963521050026,0.));
#34396=DIRECTION('center_axis',(0.,0.,1.));
#34397=DIRECTION('ref_axis',(-1.,0.,0.));
#34398=DIRECTION('center_axis',(0.,0.,-1.));
#34399=DIRECTION('ref_axis',(-1.,0.,0.));
#34400=DIRECTION('center_axis',(1.,0.,0.));
#34401=DIRECTION('ref_axis',(0.,1.,0.));
#34402=DIRECTION('',(0.,0.,1.));
#34403=DIRECTION('',(0.,0.,-1.));
#34404=DIRECTION('center_axis',(0.,0.,1.));
#34405=DIRECTION('ref_axis',(-0.70710678118655,0.707106781186545,0.));
#34406=DIRECTION('',(0.,0.,1.));
#34407=DIRECTION('center_axis',(0.,-1.,0.));
#34408=DIRECTION('ref_axis',(1.,0.,0.));
#34409=DIRECTION('center_axis',(0.,0.,-1.));
#34410=DIRECTION('ref_axis',(-1.83697019872103E-16,1.,0.));
#34411=DIRECTION('',(0.,0.,-1.));
#34412=DIRECTION('center_axis',(-0.770685380459105,-0.637215853809841,0.));
#34413=DIRECTION('ref_axis',(0.,0.,1.));
#34414=DIRECTION('',(-0.504717559062642,0.610434347646759,-0.610434347646759));
#34415=DIRECTION('',(0.,0.,1.));
#34416=DIRECTION('',(-0.504717559062642,0.610434347646759,0.610434347646759));
#34417=DIRECTION('center_axis',(0.,-0.707106781186548,-0.707106781186548));
#34418=DIRECTION('ref_axis',(-1.,0.,0.));
#34419=DIRECTION('',(1.,0.,0.));
#34420=DIRECTION('',(0.,-0.707106781186548,0.707106781186548));
#34421=DIRECTION('',(-1.,0.,0.));
#34422=DIRECTION('center_axis',(0.,0.,-1.));
#34423=DIRECTION('ref_axis',(1.,0.,0.));
#34424=DIRECTION('center_axis',(0.,0.,-1.));
#34425=DIRECTION('ref_axis',(1.,0.,0.));
#34426=DIRECTION('',(0.707106781186549,-8.65956056235495E-17,0.707106781186546));
#34427=DIRECTION('center_axis',(0.,0.,1.));
#34428=DIRECTION('ref_axis',(1.,0.,0.));
#34429=DIRECTION('center_axis',(0.,0.,1.));
#34430=DIRECTION('ref_axis',(1.,0.,0.));
#34431=DIRECTION('',(0.,1.,0.));
#34432=DIRECTION('center_axis',(0.,0.,1.));
#34433=DIRECTION('ref_axis',(0.70710678118655,0.707106781186545,0.));
#34434=DIRECTION('',(-1.,0.,0.));
#34435=DIRECTION('center_axis',(0.,0.,-1.));
#34436=DIRECTION('ref_axis',(0.707106781186547,-0.707106781186547,0.));
#34437=DIRECTION('',(0.,-1.,0.));
#34438=DIRECTION('center_axis',(0.,0.,1.));
#34439=DIRECTION('ref_axis',(-0.707106781186548,0.707106781186548,0.));
#34440=DIRECTION('',(-1.,0.,0.));
#34441=DIRECTION('center_axis',(0.,0.,1.));
#34442=DIRECTION('ref_axis',(0.707106781186548,0.707106781186548,0.));
#34443=DIRECTION('',(0.,1.,0.));
#34444=DIRECTION('center_axis',(0.,0.,1.));
#34445=DIRECTION('ref_axis',(0.707106781186545,-0.70710678118655,0.));
#34446=DIRECTION('',(1.,0.,0.));
#34447=DIRECTION('center_axis',(0.,0.,1.));
#34448=DIRECTION('ref_axis',(-0.70710678118655,-0.707106781186545,0.));
#34449=DIRECTION('',(0.,-1.,0.));
#34450=DIRECTION('center_axis',(0.,0.,-1.));
#34451=DIRECTION('ref_axis',(0.707106781186547,0.707106781186547,0.));
#34452=DIRECTION('center_axis',(0.,0.,-1.));
#34453=DIRECTION('ref_axis',(1.,0.,0.));
#34454=DIRECTION('center_axis',(0.,0.,1.));
#34455=DIRECTION('ref_axis',(1.,0.,0.));
#34456=DIRECTION('center_axis',(0.,0.,-1.));
#34457=DIRECTION('ref_axis',(1.,0.,0.));
#34458=DIRECTION('center_axis',(0.,0.,-1.));
#34459=DIRECTION('ref_axis',(1.,0.,0.));
#34460=DIRECTION('center_axis',(0.,0.,-1.));
#34461=DIRECTION('ref_axis',(1.,0.,0.));
#34462=DIRECTION('',(0.,0.,-1.));
#34463=DIRECTION('center_axis',(0.,0.,-1.));
#34464=DIRECTION('ref_axis',(1.,0.,0.));
#34465=DIRECTION('',(0.707106781186548,-8.65956056235493E-17,0.707106781186548));
#34466=DIRECTION('center_axis',(0.,0.,1.));
#34467=DIRECTION('ref_axis',(1.,0.,0.));
#34468=DIRECTION('center_axis',(0.,0.,-1.));
#34469=DIRECTION('ref_axis',(1.,0.,0.));
#34470=DIRECTION('center_axis',(0.,0.,-1.));
#34471=DIRECTION('ref_axis',(1.,0.,0.));
#34472=DIRECTION('',(0.,0.,-1.));
#34473=DIRECTION('center_axis',(0.,0.,-1.));
#34474=DIRECTION('ref_axis',(1.,0.,0.));
#34475=DIRECTION('',(0.707106781186548,-8.65956056235493E-17,0.707106781186548));
#34476=DIRECTION('center_axis',(0.,0.,1.));
#34477=DIRECTION('ref_axis',(1.,0.,0.));
#34478=DIRECTION('center_axis',(0.,0.,-1.));
#34479=DIRECTION('ref_axis',(1.,0.,0.));
#34480=DIRECTION('center_axis',(0.,0.,-1.));
#34481=DIRECTION('ref_axis',(1.,0.,0.));
#34482=DIRECTION('',(0.,0.,-1.));
#34483=DIRECTION('center_axis',(0.,0.,-1.));
#34484=DIRECTION('ref_axis',(0.707106781186548,0.707106781186548,0.));
#34485=DIRECTION('',(-0.707106781186548,0.,0.707106781186548));
#34486=DIRECTION('center_axis',(0.,0.,1.));
#34487=DIRECTION('ref_axis',(0.707106781186548,0.707106781186548,0.));
#34488=DIRECTION('center_axis',(-0.707106781186548,0.,-0.707106781186548));
#34489=DIRECTION('ref_axis',(-0.707106781186548,0.,0.707106781186548));
#34490=DIRECTION('',(-0.707106781186548,0.,0.707106781186548));
#34491=DIRECTION('',(0.,1.,0.));
#34492=DIRECTION('center_axis',(0.,0.,1.));
#34493=DIRECTION('ref_axis',(-0.70710678118655,-0.707106781186545,0.));
#34494=DIRECTION('',(0.,-0.707106781186548,0.707106781186548));
#34495=DIRECTION('center_axis',(0.,0.,-1.));
#34496=DIRECTION('ref_axis',(-0.70710678118655,-0.707106781186545,0.));
#34497=DIRECTION('center_axis',(0.,-0.707106781186548,-0.707106781186548));
#34498=DIRECTION('ref_axis',(-1.,0.,0.));
#34499=DIRECTION('',(1.25607396694702E-14,-0.707106781186548,0.707106781186548));
#34500=DIRECTION('',(-1.,0.,0.));
#34501=DIRECTION('center_axis',(0.,0.,1.));
#34502=DIRECTION('ref_axis',(0.707106781186545,-0.70710678118655,0.));
#34503=DIRECTION('',(0.707106781186548,0.,0.707106781186548));
#34504=DIRECTION('center_axis',(0.,0.,-1.));
#34505=DIRECTION('ref_axis',(0.707106781186545,-0.70710678118655,0.));
#34506=DIRECTION('center_axis',(0.707106781186548,0.,-0.707106781186548));
#34507=DIRECTION('ref_axis',(-0.707106781186548,0.,-0.707106781186548));
#34508=DIRECTION('',(0.707106781186548,0.,0.707106781186548));
#34509=DIRECTION('',(0.,-1.,0.));
#34510=DIRECTION('center_axis',(0.,0.,1.));
#34511=DIRECTION('ref_axis',(0.707106781186547,0.707106781186547,0.));
#34512=DIRECTION('',(0.,0.707106781186554,0.707106781186541));
#34513=DIRECTION('center_axis',(0.,0.,-1.));
#34514=DIRECTION('ref_axis',(0.707106781186548,0.707106781186548,0.));
#34515=DIRECTION('center_axis',(0.,0.707106781186548,-0.707106781186548));
#34516=DIRECTION('ref_axis',(-1.,0.,0.));
#34517=DIRECTION('',(0.,0.707106781186548,0.707106781186548));
#34518=DIRECTION('',(1.,0.,0.));
#34519=DIRECTION('center_axis',(0.,0.,1.));
#34520=DIRECTION('ref_axis',(-0.707106781186547,0.707106781186547,0.));
#34521=DIRECTION('',(-0.707106781186554,0.,0.707106781186541));
#34522=DIRECTION('center_axis',(0.,0.,-1.));
#34523=DIRECTION('ref_axis',(-0.707106781186548,0.707106781186548,0.));
#34524=DIRECTION('center_axis',(-0.707106781186548,0.,-0.707106781186548));
#34525=DIRECTION('ref_axis',(-0.707106781186548,0.,0.707106781186548));
#34526=DIRECTION('',(-0.707106781186548,0.,0.707106781186548));
#34527=DIRECTION('',(0.,1.,0.));
#34528=DIRECTION('center_axis',(0.,0.,-1.));
#34529=DIRECTION('ref_axis',(0.707106781186548,-0.707106781186548,0.));
#34530=DIRECTION('center_axis',(0.,0.,1.));
#34531=DIRECTION('ref_axis',(0.707106781186548,-0.707106781186548,0.));
#34532=DIRECTION('center_axis',(0.,-0.707106781186548,0.707106781186548));
#34533=DIRECTION('ref_axis',(1.,0.,0.));
#34534=DIRECTION('',(1.,0.,0.));
#34535=DIRECTION('',(0.,0.707106781186548,0.707106781186548));
#34536=DIRECTION('center_axis',(0.707106781186543,0.,-0.707106781186552));
#34537=DIRECTION('ref_axis',(-0.707106781186552,0.,-0.707106781186543));
#34538=DIRECTION('',(0.707106781186552,0.,0.707106781186543));
#34539=DIRECTION('',(0.,-1.,0.));
#34540=DIRECTION('',(-0.707106781186552,0.,-0.707106781186543));
#34541=DIRECTION('',(0.,1.,0.));
#34542=DIRECTION('center_axis',(0.,0.,1.));
#34543=DIRECTION('ref_axis',(0.70710678118655,0.707106781186545,0.));
#34544=DIRECTION('',(0.,0.707106781186547,0.707106781186548));
#34545=DIRECTION('center_axis',(0.,0.,-1.));
#34546=DIRECTION('ref_axis',(0.70710678118655,0.707106781186545,0.));
#34547=DIRECTION('center_axis',(0.,0.,1.));
#34548=DIRECTION('ref_axis',(0.70710678118655,0.707106781186545,0.));
#34549=DIRECTION('center_axis',(0.,0.707106781186549,-0.707106781186546));
#34550=DIRECTION('ref_axis',(-1.,0.,0.));
#34551=DIRECTION('',(0.,0.707106781186546,0.707106781186549));
#34552=DIRECTION('',(1.,0.,0.));
#34553=DIRECTION('',(-1.,0.,0.));
#34554=DIRECTION('center_axis',(0.,0.,1.));
#34555=DIRECTION('ref_axis',(-0.707106781186547,0.707106781186547,0.));
#34556=DIRECTION('',(-0.707106781186552,0.,0.707106781186543));
#34557=DIRECTION('center_axis',(0.,0.,-1.));
#34558=DIRECTION('ref_axis',(-0.707106781186548,0.707106781186548,0.));
#34559=DIRECTION('center_axis',(0.,0.,1.));
#34560=DIRECTION('ref_axis',(-0.707106781186548,0.707106781186548,0.));
#34561=DIRECTION('center_axis',(-0.707106781186543,0.,-0.707106781186552));
#34562=DIRECTION('ref_axis',(-0.707106781186552,0.,0.707106781186543));
#34563=DIRECTION('',(-0.707106781186552,0.,0.707106781186543));
#34564=DIRECTION('',(0.,1.,0.));
#34565=DIRECTION('',(0.,-1.,0.));
#34566=DIRECTION('center_axis',(0.,0.,1.));
#34567=DIRECTION('ref_axis',(-0.707106781186547,-0.707106781186547,0.));
#34568=DIRECTION('',(0.,-0.707106781186552,0.707106781186543));
#34569=DIRECTION('center_axis',(0.,0.,-1.));
#34570=DIRECTION('ref_axis',(-0.707106781186548,-0.707106781186548,0.));
#34571=DIRECTION('center_axis',(0.,0.,1.));
#34572=DIRECTION('ref_axis',(-0.707106781186548,-0.707106781186548,0.));
#34573=DIRECTION('center_axis',(0.,-0.707106781186543,-0.707106781186552));
#34574=DIRECTION('ref_axis',(-1.,0.,0.));
#34575=DIRECTION('',(0.,-0.707106781186552,0.707106781186543));
#34576=DIRECTION('',(-1.,0.,0.));
#34577=DIRECTION('',(1.,0.,0.));
#34578=DIRECTION('center_axis',(0.,0.,1.));
#34579=DIRECTION('ref_axis',(0.707106781186545,-0.70710678118655,0.));
#34580=DIRECTION('center_axis',(0.,0.,-1.));
#34581=DIRECTION('ref_axis',(0.707106781186545,-0.70710678118655,0.));
#34582=DIRECTION('center_axis',(0.,0.,1.));
#34583=DIRECTION('ref_axis',(0.707106781186545,-0.70710678118655,0.));
#34584=DIRECTION('center_axis',(0.,0.,1.));
#34585=DIRECTION('ref_axis',(-0.707106781186548,-0.707106781186548,0.));
#34586=DIRECTION('',(0.,0.,1.));
#34587=DIRECTION('center_axis',(0.,0.,1.));
#34588=DIRECTION('ref_axis',(-0.707106781186548,-0.707106781186548,0.));
#34589=DIRECTION('',(0.,0.,-1.));
#34590=DIRECTION('center_axis',(0.,-1.,0.));
#34591=DIRECTION('ref_axis',(1.,0.,0.));
#34592=DIRECTION('',(0.,0.,-1.));
#34593=DIRECTION('',(1.,0.,0.));
#34594=DIRECTION('center_axis',(0.,0.,1.));
#34595=DIRECTION('ref_axis',(0.707106781186545,-0.70710678118655,0.));
#34596=DIRECTION('',(0.,0.,1.));
#34597=DIRECTION('',(0.,0.,1.));
#34598=DIRECTION('center_axis',(0.,0.,1.));
#34599=DIRECTION('ref_axis',(0.707106781186545,-0.70710678118655,0.));
#34600=DIRECTION('center_axis',(1.,0.,0.));
#34601=DIRECTION('ref_axis',(0.,1.,0.));
#34602=DIRECTION('',(0.,0.,-1.));
#34603=DIRECTION('',(0.,0.,1.));
#34604=DIRECTION('',(0.,1.,0.));
#34605=DIRECTION('center_axis',(-1.,0.,0.));
#34606=DIRECTION('ref_axis',(0.,0.,-1.));
#34607=DIRECTION('center_axis',(-1.,0.,0.));
#34608=DIRECTION('ref_axis',(0.,0.,-1.));
#34609=DIRECTION('center_axis',(-1.,0.,0.));
#34610=DIRECTION('ref_axis',(0.,0.,-1.));
#34611=DIRECTION('center_axis',(0.,0.,1.));
#34612=DIRECTION('ref_axis',(1.,0.,0.));
#34613=DIRECTION('center_axis',(0.,0.,1.));
#34614=DIRECTION('ref_axis',(0.707106781186548,0.707106781186548,0.));
#34615=DIRECTION('center_axis',(0.,0.,-1.));
#34616=DIRECTION('ref_axis',(0.707106781186548,0.707106781186548,0.));
#34617=DIRECTION('',(0.707106781186548,0.,0.707106781186548));
#34618=DIRECTION('center_axis',(-0.707106781186548,0.,0.707106781186548));
#34619=DIRECTION('ref_axis',(0.707106781186548,0.,0.707106781186548));
#34620=DIRECTION('',(0.707106781186548,0.,0.707106781186548));
#34621=DIRECTION('',(0.,-1.,0.));
#34622=DIRECTION('center_axis',(0.,0.,-1.));
#34623=DIRECTION('ref_axis',(-0.70710678118655,-0.707106781186545,0.));
#34624=DIRECTION('center_axis',(0.,0.,1.));
#34625=DIRECTION('ref_axis',(-0.70710678118655,-0.707106781186545,0.));
#34626=DIRECTION('',(0.,0.707106781186548,0.707106781186548));
#34627=DIRECTION('center_axis',(0.,-0.707106781186548,0.707106781186548));
#34628=DIRECTION('ref_axis',(1.,0.,0.));
#34629=DIRECTION('',(-1.25607396694702E-14,0.707106781186548,0.707106781186548));
#34630=DIRECTION('',(1.,0.,0.));
#34631=DIRECTION('center_axis',(0.,0.,-1.));
#34632=DIRECTION('ref_axis',(0.707106781186545,-0.70710678118655,0.));
#34633=DIRECTION('center_axis',(0.,0.,1.));
#34634=DIRECTION('ref_axis',(0.707106781186545,-0.70710678118655,0.));
#34635=DIRECTION('',(-0.707106781186548,0.,0.707106781186548));
#34636=DIRECTION('center_axis',(0.707106781186548,0.,0.707106781186548));
#34637=DIRECTION('ref_axis',(0.707106781186548,0.,-0.707106781186548));
#34638=DIRECTION('',(-0.707106781186548,0.,0.707106781186548));
#34639=DIRECTION('',(0.,1.,0.));
#34640=DIRECTION('center_axis',(0.,0.,-1.));
#34641=DIRECTION('ref_axis',(0.707106781186547,0.707106781186547,0.));
#34642=DIRECTION('center_axis',(0.,0.,1.));
#34643=DIRECTION('ref_axis',(0.707106781186548,0.707106781186548,0.));
#34644=DIRECTION('',(0.,-0.707106781186554,0.707106781186541));
#34645=DIRECTION('center_axis',(0.,0.707106781186548,0.707106781186548));
#34646=DIRECTION('ref_axis',(1.,0.,0.));
#34647=DIRECTION('',(0.,-0.707106781186548,0.707106781186548));
#34648=DIRECTION('',(-1.,0.,0.));
#34649=DIRECTION('center_axis',(0.,0.,-1.));
#34650=DIRECTION('ref_axis',(-0.707106781186547,0.707106781186547,0.));
#34651=DIRECTION('center_axis',(0.,0.,1.));
#34652=DIRECTION('ref_axis',(-0.707106781186548,0.707106781186548,0.));
#34653=DIRECTION('',(0.707106781186554,0.,0.707106781186541));
#34654=DIRECTION('center_axis',(-0.707106781186548,0.,0.707106781186548));
#34655=DIRECTION('ref_axis',(0.707106781186548,0.,0.707106781186548));
#34656=DIRECTION('',(0.707106781186548,0.,0.707106781186548));
#34657=DIRECTION('',(0.,-1.,0.));
#34658=DIRECTION('center_axis',(0.,0.,1.));
#34659=DIRECTION('ref_axis',(0.707106781186548,-0.707106781186548,0.));
#34660=DIRECTION('center_axis',(0.,0.,-1.));
#34661=DIRECTION('ref_axis',(0.707106781186548,-0.707106781186548,0.));
#34662=DIRECTION('',(0.,-0.707106781186554,0.707106781186541));
#34663=DIRECTION('center_axis',(0.,0.707106781186548,0.707106781186548));
#34664=DIRECTION('ref_axis',(1.,0.,0.));
#34665=DIRECTION('',(0.,-0.707106781186548,0.707106781186548));
#34666=DIRECTION('',(-1.,0.,0.));
#34667=DIRECTION('center_axis',(0.,0.,-1.));
#34668=DIRECTION('ref_axis',(-0.707106781186547,0.707106781186547,0.));
#34669=DIRECTION('center_axis',(0.,0.,1.));
#34670=DIRECTION('ref_axis',(-0.707106781186548,0.707106781186548,0.));
#34671=DIRECTION('',(0.707106781186554,0.,0.707106781186541));
#34672=DIRECTION('center_axis',(-0.707106781186541,0.,0.707106781186554));
#34673=DIRECTION('ref_axis',(0.707106781186554,0.,0.707106781186541));
#34674=DIRECTION('',(0.707106781186554,0.,0.707106781186541));
#34675=DIRECTION('',(0.,-1.,0.));
#34676=DIRECTION('center_axis',(0.,0.,-1.));
#34677=DIRECTION('ref_axis',(-0.707106781186547,-0.707106781186547,0.));
#34678=DIRECTION('',(0.,0.707106781186554,0.707106781186541));
#34679=DIRECTION('center_axis',(0.,-0.707106781186541,0.707106781186554));
#34680=DIRECTION('ref_axis',(1.,0.,0.));
#34681=DIRECTION('',(0.,0.707106781186554,0.707106781186541));
#34682=DIRECTION('center_axis',(0.,0.,-1.));
#34683=DIRECTION('ref_axis',(0.707106781186545,-0.70710678118655,0.));
#34684=DIRECTION('',(-0.707106781186541,0.,0.707106781186554));
#34685=DIRECTION('center_axis',(0.707106781186548,0.,0.707106781186548));
#34686=DIRECTION('ref_axis',(0.707106781186548,0.,-0.707106781186548));
#34687=DIRECTION('center_axis',(-1.,0.,0.));
#34688=DIRECTION('ref_axis',(0.,-1.,0.));
#34689=DIRECTION('',(0.,0.,1.));
#34690=DIRECTION('center_axis',(0.,0.,1.));
#34691=DIRECTION('ref_axis',(-0.707106781186548,0.707106781186548,0.));
#34692=DIRECTION('',(0.,0.,-1.));
#34693=DIRECTION('center_axis',(0.,1.,0.));
#34694=DIRECTION('ref_axis',(-1.,0.,0.));
#34695=DIRECTION('',(0.,0.,1.));
#34696=DIRECTION('',(0.,0.,1.));
#34697=DIRECTION('center_axis',(0.,0.,1.));
#34698=DIRECTION('ref_axis',(0.707106781186548,-0.707106781186548,0.));
#34699=DIRECTION('',(0.,0.,-1.));
#34700=DIRECTION('center_axis',(-1.,0.,0.));
#34701=DIRECTION('ref_axis',(0.,-1.,0.));
#34702=DIRECTION('',(0.,0.,1.));
#34703=DIRECTION('center_axis',(0.,0.,1.));
#34704=DIRECTION('ref_axis',(-0.707106781186548,0.707106781186548,0.));
#34705=DIRECTION('',(0.,0.,-1.));
#34706=DIRECTION('center_axis',(0.,1.,0.));
#34707=DIRECTION('ref_axis',(-1.,0.,0.));
#34708=DIRECTION('',(0.,0.,1.));
#34709=DIRECTION('center_axis',(0.,0.,1.));
#34710=DIRECTION('ref_axis',(0.707106781186548,0.707106781186548,0.));
#34711=DIRECTION('',(0.,0.,-1.));
#34712=DIRECTION('center_axis',(1.,0.,0.));
#34713=DIRECTION('ref_axis',(0.,1.,0.));
#34714=DIRECTION('',(0.,0.,1.));
#34715=DIRECTION('center_axis',(0.,0.,1.));
#34716=DIRECTION('ref_axis',(0.707106781186545,-0.70710678118655,0.));
#34717=DIRECTION('',(0.,0.,-1.));
#34718=DIRECTION('center_axis',(0.,-1.,0.));
#34719=DIRECTION('ref_axis',(1.,0.,0.));
#34720=DIRECTION('',(0.,0.,1.));
#34721=DIRECTION('center_axis',(0.,0.,1.));
#34722=DIRECTION('ref_axis',(-0.70710678118655,-0.707106781186545,0.));
#34723=DIRECTION('',(0.,0.,-1.));
#34724=DIRECTION('center_axis',(-1.,0.,0.));
#34725=DIRECTION('ref_axis',(0.,-1.,0.));
#34726=DIRECTION('',(0.,0.,1.));
#34727=DIRECTION('center_axis',(0.,0.,1.));
#34728=DIRECTION('ref_axis',(0.707106781186548,0.707106781186548,0.));
#34729=DIRECTION('',(0.,0.,-1.));
#34730=DIRECTION('center_axis',(0.,-1.,0.));
#34731=DIRECTION('ref_axis',(1.,0.,0.));
#34732=DIRECTION('center_axis',(0.,0.,1.));
#34733=DIRECTION('ref_axis',(1.,0.,0.));
#34734=DIRECTION('',(0.707106781186548,8.65956056235493E-17,-0.707106781186548));
#34735=DIRECTION('center_axis',(0.,0.,1.));
#34736=DIRECTION('ref_axis',(1.,0.,0.));
#34737=DIRECTION('',(0.707106781186548,8.65956056235493E-17,-0.707106781186548));
#34738=DIRECTION('center_axis',(0.,0.,1.));
#34739=DIRECTION('ref_axis',(1.,0.,0.));
#34740=DIRECTION('',(0.707106781186549,8.65956056235495E-17,-0.707106781186546));
#34741=DIRECTION('center_axis',(0.,0.,1.));
#34742=DIRECTION('ref_axis',(1.,0.,0.));
#34743=DIRECTION('',(0.707106781186547,8.65956056235492E-17,-0.707106781186548));
#34744=DIRECTION('center_axis',(0.,0.,-1.));
#34745=DIRECTION('ref_axis',(1.,0.,0.));
#34746=DIRECTION('center_axis',(0.,0.,-1.));
#34747=DIRECTION('ref_axis',(1.,0.,0.));
#34748=DIRECTION('',(0.,0.,-1.));
#34749=DIRECTION('center_axis',(0.,0.,-1.));
#34750=DIRECTION('ref_axis',(1.,0.,0.));
#34751=DIRECTION('',(0.,0.,-1.));
#34752=DIRECTION('center_axis',(0.,0.,-1.));
#34753=DIRECTION('ref_axis',(1.,0.,0.));
#34754=DIRECTION('',(0.,0.,-1.));
#34755=DIRECTION('center_axis',(0.,0.,-1.));
#34756=DIRECTION('ref_axis',(1.,0.,0.));
#34757=DIRECTION('center_axis',(0.,0.,1.));
#34758=DIRECTION('ref_axis',(1.,0.,0.));
#34759=DIRECTION('center_axis',(-1.,0.,0.));
#34760=DIRECTION('ref_axis',(0.,0.,-1.));
#34761=DIRECTION('',(-1.,0.,0.));
#34762=DIRECTION('',(-1.,0.,0.));
#34763=DIRECTION('center_axis',(-1.,0.,0.));
#34764=DIRECTION('ref_axis',(0.,0.,-1.));
#34765=DIRECTION('center_axis',(1.,0.,0.));
#34766=DIRECTION('ref_axis',(0.,0.,-1.));
#34767=DIRECTION('center_axis',(-1.,0.,0.));
#34768=DIRECTION('ref_axis',(0.,0.,-1.));
#34769=DIRECTION('',(-1.,0.,0.));
#34770=DIRECTION('center_axis',(-1.,0.,0.));
#34771=DIRECTION('ref_axis',(0.,0.,-1.));
#34772=DIRECTION('center_axis',(1.,0.,0.));
#34773=DIRECTION('ref_axis',(0.,0.,-1.));
#34774=DIRECTION('center_axis',(0.,0.,1.));
#34775=DIRECTION('ref_axis',(1.,0.,0.));
#34776=DIRECTION('center_axis',(0.,0.,1.));
#34777=DIRECTION('ref_axis',(1.,0.,0.));
#34778=DIRECTION('center_axis',(0.,0.,-1.));
#34779=DIRECTION('ref_axis',(1.,0.,0.));
#34780=DIRECTION('',(0.,0.,-1.));
#34781=DIRECTION('center_axis',(0.,0.,-1.));
#34782=DIRECTION('ref_axis',(1.,0.,0.));
#34783=DIRECTION('center_axis',(0.,0.,1.));
#34784=DIRECTION('ref_axis',(1.,0.,0.));
#34785=DIRECTION('center_axis',(0.,0.,-1.));
#34786=DIRECTION('ref_axis',(1.,0.,0.));
#34787=DIRECTION('',(0.,0.,-1.));
#34788=DIRECTION('center_axis',(0.,0.,-1.));
#34789=DIRECTION('ref_axis',(1.,0.,0.));
#34790=DIRECTION('center_axis',(0.,0.,1.));
#34791=DIRECTION('ref_axis',(1.,0.,0.));
#34792=DIRECTION('center_axis',(0.,0.,-1.));
#34793=DIRECTION('ref_axis',(1.,0.,0.));
#34794=DIRECTION('',(0.,0.,-1.));
#34795=DIRECTION('center_axis',(0.,0.,-1.));
#34796=DIRECTION('ref_axis',(1.,0.,0.));
#34797=DIRECTION('center_axis',(0.,0.,1.));
#34798=DIRECTION('ref_axis',(1.,0.,0.));
#34799=DIRECTION('center_axis',(0.,0.,1.));
#34800=DIRECTION('ref_axis',(0.707106781186545,-0.70710678118655,0.));
#34801=DIRECTION('',(0.,0.,-1.));
#34802=DIRECTION('center_axis',(0.,-1.,0.));
#34803=DIRECTION('ref_axis',(1.,0.,0.));
#34804=DIRECTION('center_axis',(0.,0.,1.));
#34805=DIRECTION('ref_axis',(0.70710678118655,0.707106781186545,0.));
#43120=CARTESIAN_POINT('',(0.,0.,0.));
#43121=CARTESIAN_POINT('Origin',(-56.25,18.75,29.075));
#43122=CARTESIAN_POINT('',(-58.8,18.75,29.325));
#43123=CARTESIAN_POINT('Origin',(-56.25,18.75,29.325));
#43124=CARTESIAN_POINT('',(-58.3,18.75,28.825));
#43125=CARTESIAN_POINT('',(-58.55,18.75,29.075));
#43126=CARTESIAN_POINT('Origin',(-56.25,18.75,28.825));
#43127=CARTESIAN_POINT('Origin',(0.,0.,29.325));
#43128=CARTESIAN_POINT('',(-54.5,-58.,29.325));
#43129=CARTESIAN_POINT('',(-54.5,-82.5,29.325));
#43130=CARTESIAN_POINT('',(-54.5,-35.,29.325));
#43131=CARTESIAN_POINT('',(-49.,-58.,29.325));
#43132=CARTESIAN_POINT('',(-27.,-58.,29.325));
#43133=CARTESIAN_POINT('',(-46.5,-55.5,29.325));
#43134=CARTESIAN_POINT('Origin',(-49.,-55.5,29.325));
#43135=CARTESIAN_POINT('',(-46.5,-43.,29.325));
#43136=CARTESIAN_POINT('',(-46.5,-29.25,29.325));
#43137=CARTESIAN_POINT('',(-43.,-39.5,29.325));
#43138=CARTESIAN_POINT('Origin',(-43.,-43.,29.325));
#43139=CARTESIAN_POINT('',(-12.3389626792531,-39.5,29.325));
#43140=CARTESIAN_POINT('',(-23.,-39.5,29.325));
#43141=CARTESIAN_POINT('',(12.3389626792531,-39.5,29.325));
#43142=CARTESIAN_POINT('Origin',(0.,-37.5,29.325));
#43143=CARTESIAN_POINT('',(39.,-39.5,29.325));
#43144=CARTESIAN_POINT('',(-23.,-39.5,29.325));
#43145=CARTESIAN_POINT('',(42.5,-43.,29.325));
#43146=CARTESIAN_POINT('Origin',(39.,-43.,29.325));
#43147=CARTESIAN_POINT('',(42.5,-67.,29.325));
#43148=CARTESIAN_POINT('',(42.5,-20.,29.325));
#43149=CARTESIAN_POINT('',(45.,-69.5,29.325));
#43150=CARTESIAN_POINT('Origin',(45.,-67.,29.325));
#43151=CARTESIAN_POINT('',(67.,-69.5,29.325));
#43152=CARTESIAN_POINT('',(21.,-69.5,29.325));
#43153=CARTESIAN_POINT('',(69.5,-67.,29.325));
#43154=CARTESIAN_POINT('Origin',(67.,-67.,29.325));
#43155=CARTESIAN_POINT('',(69.5,67.,29.325));
#43156=CARTESIAN_POINT('',(69.5,-35.,29.325));
#43157=CARTESIAN_POINT('',(67.,69.5,29.325));
#43158=CARTESIAN_POINT('Origin',(67.,67.,29.325));
#43159=CARTESIAN_POINT('',(-67.,69.5,29.325));
#43160=CARTESIAN_POINT('',(35.,69.5,29.325));
#43161=CARTESIAN_POINT('',(-69.5,67.,29.325));
#43162=CARTESIAN_POINT('Origin',(-67.,67.,29.325));
#43163=CARTESIAN_POINT('',(-69.5,-51.,29.325));
#43164=CARTESIAN_POINT('',(-69.5,35.,29.325));
#43165=CARTESIAN_POINT('',(-73.,-54.5,29.325));
#43166=CARTESIAN_POINT('Origin',(-73.,-51.,29.325));
#43167=CARTESIAN_POINT('',(-81.,-54.5,29.325));
#43168=CARTESIAN_POINT('',(-27.,-54.5,29.325));
#43169=CARTESIAN_POINT('',(-83.5,-57.,29.325));
#43170=CARTESIAN_POINT('Origin',(-81.,-57.,29.325));
#43171=CARTESIAN_POINT('',(-83.5,-82.5,29.325));
#43172=CARTESIAN_POINT('',(-83.5,-27.,29.325));
#43173=CARTESIAN_POINT('',(-81.,-85.,29.325));
#43174=CARTESIAN_POINT('Origin',(-81.,-82.5,29.325));
#43175=CARTESIAN_POINT('',(-57.,-85.,29.325));
#43176=CARTESIAN_POINT('',(-42.,-85.,29.325));
#43177=CARTESIAN_POINT('Origin',(-57.,-82.5,29.325));
#43178=CARTESIAN_POINT('',(-21.3,56.25,29.325));
#43179=CARTESIAN_POINT('Origin',(-18.75,56.25,29.325));
#43180=CARTESIAN_POINT('',(25.,-1.53080849893419E-15,29.325));
#43181=CARTESIAN_POINT('Origin',(37.5,0.,29.325));
#43182=CARTESIAN_POINT('',(-12.5,37.5,29.325));
#43183=CARTESIAN_POINT('Origin',(0.,37.5,29.325));
#43184=CARTESIAN_POINT('',(-61.5,-79.,29.325));
#43185=CARTESIAN_POINT('Origin',(-60.,-79.,29.325));
#43186=CARTESIAN_POINT('',(47.425,52.425,29.325));
#43187=CARTESIAN_POINT('Origin',(52.425,52.425,29.325));
#43188=CARTESIAN_POINT('',(-57.425,-52.425,29.325));
#43189=CARTESIAN_POINT('Origin',(-52.425,-52.425,29.325));
#43190=CARTESIAN_POINT('',(-56.6629,52.425,29.325));
#43191=CARTESIAN_POINT('Origin',(-52.425,52.425,29.325));
#43192=CARTESIAN_POINT('',(-5.625,-6.88863824520386E-16,29.325));
#43193=CARTESIAN_POINT('Origin',(0.,0.,29.325));
#43194=CARTESIAN_POINT('',(-50.,-1.53080849893419E-15,29.325));
#43195=CARTESIAN_POINT('Origin',(-37.5,0.,29.325));
#43196=CARTESIAN_POINT('Origin',(-56.25,18.75,29.325));
#43197=CARTESIAN_POINT('',(-58.3,18.75,20.825));
#43198=CARTESIAN_POINT('',(-58.3,18.75,29.325));
#43199=CARTESIAN_POINT('Origin',(-56.25,18.75,20.825));
#43200=CARTESIAN_POINT('Origin',(-18.75,56.25,29.075));
#43201=CARTESIAN_POINT('',(-20.8,56.25,28.825));
#43202=CARTESIAN_POINT('',(-21.05,56.25,29.075));
#43203=CARTESIAN_POINT('Origin',(-18.75,56.25,28.825));
#43204=CARTESIAN_POINT('Origin',(-18.75,56.25,29.325));
#43205=CARTESIAN_POINT('',(-20.8,56.25,20.825));
#43206=CARTESIAN_POINT('',(-20.8,56.25,29.325));
#43207=CARTESIAN_POINT('Origin',(-18.75,56.25,20.825));
#43208=CARTESIAN_POINT('Origin',(-27.,-58.25,29.075));
#43209=CARTESIAN_POINT('',(-54.,-58.5,28.825));
#43210=CARTESIAN_POINT('',(-53.5833333333333,-58.9166666666667,28.4083333333333));
#43211=CARTESIAN_POINT('',(-49.,-58.5,28.825));
#43212=CARTESIAN_POINT('',(-27.,-58.5,28.825));
#43213=CARTESIAN_POINT('',(-49.,-58.5,28.825));
#43214=CARTESIAN_POINT('Origin',(-49.,-55.5,29.075));
#43215=CARTESIAN_POINT('',(-46.,-55.5,28.825));
#43216=CARTESIAN_POINT('Origin',(-49.,-55.5,28.825));
#43217=CARTESIAN_POINT('',(-46.,-55.5,28.825));
#43218=CARTESIAN_POINT('Origin',(-46.25,-29.25,29.075));
#43219=CARTESIAN_POINT('',(-46.,-43.,28.825));
#43220=CARTESIAN_POINT('',(-46.,-43.,28.825));
#43221=CARTESIAN_POINT('',(-46.,-29.25,28.825));
#43222=CARTESIAN_POINT('Origin',(-43.,-43.,29.075));
#43223=CARTESIAN_POINT('',(-43.,-40.,28.825));
#43224=CARTESIAN_POINT('Origin',(-43.,-43.,28.825));
#43225=CARTESIAN_POINT('',(-43.,-40.,28.825));
#43226=CARTESIAN_POINT('Origin',(-23.,-39.75,29.075));
#43227=CARTESIAN_POINT('',(-12.034713649895,-39.7557126677597,29.0692873322403));
#43228=CARTESIAN_POINT('Ctrl Pts',(-12.034713649895,-39.7557126677597,29.0692873322403));
#43229=CARTESIAN_POINT('Ctrl Pts',(-12.186838165433,-39.6294523240611,29.1955476759389));
#43230=CARTESIAN_POINT('Ctrl Pts',(-12.3389626809711,-39.499999998538,29.325000001462));
#43231=CARTESIAN_POINT('',(-12.2366945943055,-40.,28.825));
#43232=CARTESIAN_POINT('',(-23.,-40.,28.825));
#43233=CARTESIAN_POINT('',(-13.3898823845721,-41.3947314172564,27.4302685827436));
#43234=CARTESIAN_POINT('Origin',(0.,-37.5,29.075));
#43235=CARTESIAN_POINT('',(-11.8306505499589,-39.508907057272,28.825));
#43236=CARTESIAN_POINT('Ctrl Pts',(-11.8306505487286,-39.5089070557841,
28.824999998538));
#43237=CARTESIAN_POINT('Ctrl Pts',(-11.9316540214349,-39.6310664454554,
28.9450286360224));
#43238=CARTESIAN_POINT('Ctrl Pts',(-12.034713649895,-39.7557126677596,29.0692873322403));
#43239=CARTESIAN_POINT('',(11.8306505499589,-39.508907057272,28.825));
#43240=CARTESIAN_POINT('Origin',(0.,-37.5,28.825));
#43241=CARTESIAN_POINT('',(12.0347136500218,-39.755712667654,29.0692873324511));
#43242=CARTESIAN_POINT('Ctrl Pts',(12.0347136500218,-39.755712667654,29.0692873324511));
#43243=CARTESIAN_POINT('Ctrl Pts',(11.9316540215288,-39.6310664453101,28.9450286361929));
#43244=CARTESIAN_POINT('Ctrl Pts',(11.8306505487286,-39.5089070557841,28.824999998538));
#43245=CARTESIAN_POINT('Ctrl Pts',(12.3389626792531,-39.5,29.325));
#43246=CARTESIAN_POINT('Ctrl Pts',(12.2383051553503,-39.5856558228154,29.2393441771846));
#43247=CARTESIAN_POINT('Ctrl Pts',(12.1368860140384,-39.6709116232476,29.1540883767524));
#43248=CARTESIAN_POINT('Ctrl Pts',(12.0347136501489,-39.7557126675489,29.0692873324511));
#43249=CARTESIAN_POINT('Origin',(-12.0336725721322,-39.754453528636,29.325));
#43250=CARTESIAN_POINT('',(-12.2366945943055,-40.,20.3));
#43251=CARTESIAN_POINT('',(-12.2366945943055,-40.,29.325));
#43252=CARTESIAN_POINT('',(-11.8306505499589,-39.508907057272,20.3));
#43253=CARTESIAN_POINT('',(-12.2366945943055,-40.,20.3));
#43254=CARTESIAN_POINT('',(-11.8306505499589,-39.508907057272,29.325));
#43255=CARTESIAN_POINT('Origin',(-11.8306505499589,-39.508907057272,20.3));
#43256=CARTESIAN_POINT('',(-12.3389626792531,-39.5,19.8));
#43257=CARTESIAN_POINT('Ctrl Pts',(-12.338962679254,-39.5,19.7999999999991));
#43258=CARTESIAN_POINT('Ctrl Pts',(-12.0805946952053,-39.5047062025856,
20.0542864406007));
#43259=CARTESIAN_POINT('Ctrl Pts',(-11.8306505499589,-39.508907057272,20.3));
#43260=CARTESIAN_POINT('',(-12.3389626792531,-39.5,19.8));
#43261=CARTESIAN_POINT('Origin',(-27.,-58.25,20.05));
#43262=CARTESIAN_POINT('',(-54.,-58.5,20.3));
#43263=CARTESIAN_POINT('',(-54.,-58.,19.8));
#43264=CARTESIAN_POINT('',(-54.,-61.125,22.925));
#43265=CARTESIAN_POINT('',(-49.,-58.,19.8));
#43266=CARTESIAN_POINT('',(-27.,-58.,19.8));
#43267=CARTESIAN_POINT('',(-49.,-58.5,20.3));
#43268=CARTESIAN_POINT('',(-49.,-58.,19.8));
#43269=CARTESIAN_POINT('',(-27.,-58.5,20.3));
#43270=CARTESIAN_POINT('Origin',(-49.,-55.5,20.05));
#43271=CARTESIAN_POINT('',(-46.5,-55.5,19.8));
#43272=CARTESIAN_POINT('',(-46.,-55.5,20.3));
#43273=CARTESIAN_POINT('',(-46.5,-55.5,19.8));
#43274=CARTESIAN_POINT('Origin',(-49.,-55.5,20.3));
#43275=CARTESIAN_POINT('Origin',(-49.,-55.5,19.8));
#43276=CARTESIAN_POINT('Origin',(-46.25,-29.25,20.05));
#43277=CARTESIAN_POINT('',(-46.5,-43.,19.8));
#43278=CARTESIAN_POINT('',(-46.,-43.,20.3));
#43279=CARTESIAN_POINT('',(-46.5,-43.,19.8));
#43280=CARTESIAN_POINT('',(-46.,-29.25,20.3));
#43281=CARTESIAN_POINT('',(-46.5,-29.25,19.8));
#43282=CARTESIAN_POINT('Origin',(-43.,-43.,20.05));
#43283=CARTESIAN_POINT('',(-43.,-39.5,19.8));
#43284=CARTESIAN_POINT('',(-43.,-40.,20.3));
#43285=CARTESIAN_POINT('',(-43.,-39.5,19.8));
#43286=CARTESIAN_POINT('Origin',(-43.,-43.,20.3));
#43287=CARTESIAN_POINT('Origin',(-43.,-43.,19.8));
#43288=CARTESIAN_POINT('Origin',(-23.,-39.75,20.05));
#43289=CARTESIAN_POINT('',(-23.,-39.5,19.8));
#43290=CARTESIAN_POINT('',(-23.,-40.,20.3));
#43291=CARTESIAN_POINT('Origin',(0.,-37.5,20.05));
#43292=CARTESIAN_POINT('',(12.034713649895,-39.7557126677597,20.0557126677597));
#43293=CARTESIAN_POINT('',(11.8306505499589,-39.508907057272,20.3));
#43294=CARTESIAN_POINT('Ctrl Pts',(12.034713649895,-39.7557126677597,20.0557126677597));
#43295=CARTESIAN_POINT('Ctrl Pts',(11.9316540220625,-39.6310664462144,20.1799713632209));
#43296=CARTESIAN_POINT('Ctrl Pts',(11.8306505499589,-39.508907057272,20.3));
#43297=CARTESIAN_POINT('Origin',(0.,-37.5,20.3));
#43298=CARTESIAN_POINT('',(12.3389626792531,-39.5,19.8));
#43299=CARTESIAN_POINT('Origin',(0.,-37.5,19.8));
#43300=CARTESIAN_POINT('Ctrl Pts',(12.3389626792531,-39.5,19.8));
#43301=CARTESIAN_POINT('Ctrl Pts',(12.1868381645741,-39.6294523247741,19.929452324774));
#43302=CARTESIAN_POINT('Ctrl Pts',(12.034713649895,-39.7557126677597,20.0557126677597));
#43303=CARTESIAN_POINT('Origin',(-46.,-58.5,19.8));
#43304=CARTESIAN_POINT('',(-46.,-55.5,19.8));
#43305=CARTESIAN_POINT('',(-46.,-43.,19.8));
#43306=CARTESIAN_POINT('Origin',(-43.,-43.,19.8));
#43307=CARTESIAN_POINT('',(-43.,-40.,19.8));
#43308=CARTESIAN_POINT('Origin',(-46.,-40.,19.8));
#43309=CARTESIAN_POINT('Origin',(0.,-37.5,29.325));
#43310=CARTESIAN_POINT('',(11.8306505499589,-39.508907057272,29.325));
#43311=CARTESIAN_POINT('Origin',(12.0336725721322,-39.754453528636,29.325));
#43312=CARTESIAN_POINT('',(12.2366945943055,-40.,20.3));
#43313=CARTESIAN_POINT('',(12.2366945943055,-40.,20.3));
#43314=CARTESIAN_POINT('',(12.2366945943055,-40.,28.825));
#43315=CARTESIAN_POINT('',(12.2366945943055,-40.,29.325));
#43316=CARTESIAN_POINT('',(7.53086665277066,-34.3085019372742,34.5164980627258));
#43317=CARTESIAN_POINT('Origin',(-23.,-39.75,20.05));
#43318=CARTESIAN_POINT('',(39.,-39.5,19.8));
#43319=CARTESIAN_POINT('',(-23.,-39.5,19.8));
#43320=CARTESIAN_POINT('',(39.,-40.,20.3));
#43321=CARTESIAN_POINT('',(39.,-39.5,19.8));
#43322=CARTESIAN_POINT('',(-23.,-40.,20.3));
#43323=CARTESIAN_POINT('Origin',(0.,37.5,20.05));
#43324=CARTESIAN_POINT('',(-12.5,37.5,19.8));
#43325=CARTESIAN_POINT('Origin',(0.,37.5,19.8));
#43326=CARTESIAN_POINT('',(-12.,37.5,20.3));
#43327=CARTESIAN_POINT('',(-12.25,37.5,20.05));
#43328=CARTESIAN_POINT('Origin',(0.,37.5,20.3));
#43329=CARTESIAN_POINT('Origin',(0.,0.,19.8));
#43330=CARTESIAN_POINT('',(-54.,-57.,19.8));
#43331=CARTESIAN_POINT('',(-54.,-42.75,19.8));
#43332=CARTESIAN_POINT('',(-57.,-54.,19.8));
#43333=CARTESIAN_POINT('Origin',(-57.,-57.,19.8));
#43334=CARTESIAN_POINT('',(-71.197224362268,-54.,19.8));
#43335=CARTESIAN_POINT('',(-27.,-54.,19.8));
#43336=CARTESIAN_POINT('',(-69.5,-51.,19.8));
#43337=CARTESIAN_POINT('Origin',(-73.,-51.,19.8));
#43338=CARTESIAN_POINT('',(-69.5,67.,19.8));
#43339=CARTESIAN_POINT('',(-69.5,35.,19.8));
#43340=CARTESIAN_POINT('',(-67.,69.5,19.8));
#43341=CARTESIAN_POINT('Origin',(-67.,67.,19.8));
#43342=CARTESIAN_POINT('',(67.,69.5,19.8));
#43343=CARTESIAN_POINT('',(35.,69.5,19.8));
#43344=CARTESIAN_POINT('',(69.5,67.,19.8));
#43345=CARTESIAN_POINT('Origin',(67.,67.,19.8));
#43346=CARTESIAN_POINT('',(69.5,-67.,19.8));
#43347=CARTESIAN_POINT('',(69.5,-35.,19.8));
#43348=CARTESIAN_POINT('',(67.,-69.5,19.8));
#43349=CARTESIAN_POINT('Origin',(67.,-67.,19.8));
#43350=CARTESIAN_POINT('',(45.,-69.5,19.8));
#43351=CARTESIAN_POINT('',(21.,-69.5,19.8));
#43352=CARTESIAN_POINT('',(42.5,-67.,19.8));
#43353=CARTESIAN_POINT('Origin',(45.,-67.,19.8));
#43354=CARTESIAN_POINT('',(42.5,-43.,19.8));
#43355=CARTESIAN_POINT('',(42.5,-20.,19.8));
#43356=CARTESIAN_POINT('Origin',(39.,-43.,19.8));
#43357=CARTESIAN_POINT('',(-50.,1.53080849893419E-15,19.8));
#43358=CARTESIAN_POINT('Origin',(-37.5,0.,19.8));
#43359=CARTESIAN_POINT('',(-5.025,-6.15385016571545E-16,19.8));
#43360=CARTESIAN_POINT('Origin',(0.,0.,19.8));
#43361=CARTESIAN_POINT('',(25.,1.53080849893419E-15,19.8));
#43362=CARTESIAN_POINT('Origin',(37.5,0.,19.8));
#43363=CARTESIAN_POINT('Origin',(0.,37.5,29.325));
#43364=CARTESIAN_POINT('',(-12.,37.5,28.825));
#43365=CARTESIAN_POINT('Origin',(0.,37.5,28.825));
#43366=CARTESIAN_POINT('',(-12.,37.5,29.325));
#43367=CARTESIAN_POINT('Origin',(-37.5,0.,20.05));
#43368=CARTESIAN_POINT('',(-49.5,-1.46957615897682E-15,20.3));
#43369=CARTESIAN_POINT('',(-49.75,1.50019232895551E-15,20.05));
#43370=CARTESIAN_POINT('Origin',(-37.5,0.,20.3));
#43371=CARTESIAN_POINT('Origin',(-37.5,0.,29.325));
#43372=CARTESIAN_POINT('',(-49.5,1.46957615897682E-15,28.825));
#43373=CARTESIAN_POINT('Origin',(-37.5,0.,28.825));
#43374=CARTESIAN_POINT('',(-49.5,1.46957615897682E-15,29.325));
#43375=CARTESIAN_POINT('Origin',(37.5,0.,20.05));
#43376=CARTESIAN_POINT('',(25.5,-1.46957615897682E-15,20.3));
#43377=CARTESIAN_POINT('',(25.25,1.50019232895551E-15,20.05));
#43378=CARTESIAN_POINT('Origin',(37.5,0.,20.3));
#43379=CARTESIAN_POINT('Origin',(37.5,0.,29.325));
#43380=CARTESIAN_POINT('',(25.5,1.46957615897682E-15,28.825));
#43381=CARTESIAN_POINT('Origin',(37.5,0.,28.825));
#43382=CARTESIAN_POINT('',(25.5,1.46957615897682E-15,29.325));
#43383=CARTESIAN_POINT('Origin',(39.,-43.,20.05));
#43384=CARTESIAN_POINT('',(42.,-43.,20.3));
#43385=CARTESIAN_POINT('',(42.5,-43.,19.8));
#43386=CARTESIAN_POINT('Origin',(39.,-43.,20.3));
#43387=CARTESIAN_POINT('Origin',(42.25,-20.,20.05));
#43388=CARTESIAN_POINT('',(42.,-67.,20.3));
#43389=CARTESIAN_POINT('',(42.5,-67.,19.8));
#43390=CARTESIAN_POINT('',(42.,-20.,20.3));
#43391=CARTESIAN_POINT('Origin',(45.,-67.,20.05));
#43392=CARTESIAN_POINT('',(45.,-70.,20.3));
#43393=CARTESIAN_POINT('',(45.,-69.5,19.8));
#43394=CARTESIAN_POINT('Origin',(45.,-67.,20.3));
#43395=CARTESIAN_POINT('Origin',(21.,-69.75,20.05));
#43396=CARTESIAN_POINT('',(67.,-70.,20.3));
#43397=CARTESIAN_POINT('',(67.,-69.5,19.8));
#43398=CARTESIAN_POINT('',(21.,-70.,20.3));
#43399=CARTESIAN_POINT('Origin',(67.,-67.,20.05));
#43400=CARTESIAN_POINT('',(70.,-67.,20.3));
#43401=CARTESIAN_POINT('',(69.5,-67.,19.8));
#43402=CARTESIAN_POINT('Origin',(67.,-67.,20.3));
#43403=CARTESIAN_POINT('Origin',(69.75,-35.,20.05));
#43404=CARTESIAN_POINT('',(70.,67.,20.3));
#43405=CARTESIAN_POINT('',(69.5,67.,19.8));
#43406=CARTESIAN_POINT('',(70.,-35.,20.3));
#43407=CARTESIAN_POINT('Origin',(67.,67.,20.05));
#43408=CARTESIAN_POINT('',(67.,70.,20.3));
#43409=CARTESIAN_POINT('',(67.,69.5,19.8));
#43410=CARTESIAN_POINT('Origin',(67.,67.,20.3));
#43411=CARTESIAN_POINT('Origin',(35.,69.75,20.05));
#43412=CARTESIAN_POINT('',(-67.,70.,20.3));
#43413=CARTESIAN_POINT('',(-67.,69.5,19.8));
#43414=CARTESIAN_POINT('',(35.,70.,20.3));
#43415=CARTESIAN_POINT('Origin',(-67.,67.,20.05));
#43416=CARTESIAN_POINT('',(-70.,67.,20.3));
#43417=CARTESIAN_POINT('',(-69.5,67.,19.8));
#43418=CARTESIAN_POINT('Origin',(-67.,67.,20.3));
#43419=CARTESIAN_POINT('Origin',(-69.75,35.,20.05));
#43420=CARTESIAN_POINT('',(-70.,-51.,20.3));
#43421=CARTESIAN_POINT('',(-69.5,-51.,19.8));
#43422=CARTESIAN_POINT('',(-70.,35.,20.3));
#43423=CARTESIAN_POINT('Origin',(-73.,-51.,20.05));
#43424=CARTESIAN_POINT('',(-73.,-54.,20.3));
#43425=CARTESIAN_POINT('Ctrl Pts',(-73.,-54.,20.3));
#43426=CARTESIAN_POINT('Ctrl Pts',(-72.1679497056621,-54.,20.3));
#43427=CARTESIAN_POINT('Ctrl Pts',(-71.197224362268,-54.,19.8));
#43428=CARTESIAN_POINT('Origin',(-73.,-51.,20.3));
#43429=CARTESIAN_POINT('Origin',(-23.,-39.75,29.075));
#43430=CARTESIAN_POINT('',(39.,-40.,28.825));
#43431=CARTESIAN_POINT('',(-23.,-40.,28.825));
#43432=CARTESIAN_POINT('',(39.,-40.,28.825));
#43433=CARTESIAN_POINT('Origin',(-54.25,-69.875,1.25));
#43434=CARTESIAN_POINT('',(-54.5,-57.,1.));
#43435=CARTESIAN_POINT('',(-54.,-57.,1.5));
#43436=CARTESIAN_POINT('',(-54.5,-57.,1.));
#43437=CARTESIAN_POINT('',(-54.,-82.5,1.5));
#43438=CARTESIAN_POINT('',(-54.,-69.875,1.5));
#43439=CARTESIAN_POINT('',(-54.5,-82.5,1.));
#43440=CARTESIAN_POINT('',(-54.,-82.5,1.5));
#43441=CARTESIAN_POINT('',(-54.5,-69.875,1.));
#43442=CARTESIAN_POINT('Origin',(-57.,-57.,1.25));
#43443=CARTESIAN_POINT('',(-57.,-54.5,1.));
#43444=CARTESIAN_POINT('',(-57.,-54.,1.5));
#43445=CARTESIAN_POINT('',(-57.,-54.5,1.));
#43446=CARTESIAN_POINT('Origin',(-57.,-57.,1.5));
#43447=CARTESIAN_POINT('Origin',(-57.,-57.,1.));
#43448=CARTESIAN_POINT('Origin',(-61.5,-54.25,1.25));
#43449=CARTESIAN_POINT('',(-81.,-54.5,1.));
#43450=CARTESIAN_POINT('',(-81.,-54.,1.5));
#43451=CARTESIAN_POINT('',(-81.,-54.5,1.));
#43452=CARTESIAN_POINT('',(-61.5,-54.,1.5));
#43453=CARTESIAN_POINT('',(-61.5,-54.5,1.));
#43454=CARTESIAN_POINT('Origin',(-81.,-57.,1.25));
#43455=CARTESIAN_POINT('',(-83.5,-57.,1.));
#43456=CARTESIAN_POINT('',(-84.,-57.,1.5));
#43457=CARTESIAN_POINT('',(-83.5,-57.,1.));
#43458=CARTESIAN_POINT('Origin',(-81.,-57.,1.5));
#43459=CARTESIAN_POINT('Origin',(-81.,-57.,1.));
#43460=CARTESIAN_POINT('Origin',(-83.75,-61.875,1.25));
#43461=CARTESIAN_POINT('',(-83.5,-82.5,1.));
#43462=CARTESIAN_POINT('',(-84.,-82.5,1.5));
#43463=CARTESIAN_POINT('',(-83.5,-82.5,1.));
#43464=CARTESIAN_POINT('',(-84.,-61.875,1.5));
#43465=CARTESIAN_POINT('',(-83.5,-61.875,1.));
#43466=CARTESIAN_POINT('Origin',(-81.,-82.5,1.25));
#43467=CARTESIAN_POINT('',(-81.,-85.,1.));
#43468=CARTESIAN_POINT('',(-81.,-85.5,1.5));
#43469=CARTESIAN_POINT('',(-81.,-85.,1.));
#43470=CARTESIAN_POINT('Origin',(-81.,-82.5,1.5));
#43471=CARTESIAN_POINT('Origin',(-81.,-82.5,1.));
#43472=CARTESIAN_POINT('Origin',(-76.5,-85.25,1.25));
#43473=CARTESIAN_POINT('',(-57.,-85.,1.));
#43474=CARTESIAN_POINT('',(-57.,-85.5,1.5));
#43475=CARTESIAN_POINT('',(-57.,-85.,1.));
#43476=CARTESIAN_POINT('',(-76.5,-85.5,1.5));
#43477=CARTESIAN_POINT('',(-76.5,-85.,1.));
#43478=CARTESIAN_POINT('Origin',(-57.,-82.5,1.25));
#43479=CARTESIAN_POINT('Origin',(-57.,-82.5,1.5));
#43480=CARTESIAN_POINT('Origin',(-57.,-82.5,1.));
#43481=CARTESIAN_POINT('Origin',(-81.,-82.5,1.));
#43482=CARTESIAN_POINT('',(-81.,-85.5,28.825));
#43483=CARTESIAN_POINT('',(-81.,-85.5,1.));
#43484=CARTESIAN_POINT('',(-84.,-82.5,28.825));
#43485=CARTESIAN_POINT('Origin',(-81.,-82.5,28.825));
#43486=CARTESIAN_POINT('',(-84.,-82.5,1.));
#43487=CARTESIAN_POINT('Origin',(-84.,-85.5,1.));
#43488=CARTESIAN_POINT('',(-57.,-85.5,28.825));
#43489=CARTESIAN_POINT('',(-57.,-85.5,10.4));
#43490=CARTESIAN_POINT('',(-42.,-85.5,28.825));
#43491=CARTESIAN_POINT('Origin',(-57.,-82.5,10.4));
#43492=CARTESIAN_POINT('',(-54.,-82.5,17.1715728752538));
#43493=CARTESIAN_POINT('',(-54.,-82.5,10.4));
#43494=CARTESIAN_POINT('',(-54.,-82.5,22.8284271247462));
#43495=CARTESIAN_POINT('Ctrl Pts',(-54.,-82.5,17.1715728752538));
#43496=CARTESIAN_POINT('Ctrl Pts',(-54.,-82.762296060057,17.4961476900572));
#43497=CARTESIAN_POINT('Ctrl Pts',(-54.034665028442,-82.985258794199,17.8667160823623));
#43498=CARTESIAN_POINT('Ctrl Pts',(-54.1231965863205,-83.3837724986897,
18.8181489326506));
#43499=CARTESIAN_POINT('Ctrl Pts',(-54.1715728752538,-83.5,19.4255653846135));
#43500=CARTESIAN_POINT('Ctrl Pts',(-54.1715728752538,-83.5,20.5744346153865));
#43501=CARTESIAN_POINT('Ctrl Pts',(-54.1231965863205,-83.3837724986897,
21.1818510673494));
#43502=CARTESIAN_POINT('Ctrl Pts',(-54.034665028442,-82.985258794199,22.1332839176377));
#43503=CARTESIAN_POINT('Ctrl Pts',(-54.,-82.762296060057,22.5038523099428));
#43504=CARTESIAN_POINT('Ctrl Pts',(-54.,-82.5,22.8284271247462));
#43505=CARTESIAN_POINT('',(-54.,-82.5,28.825));
#43506=CARTESIAN_POINT('',(-54.,-82.5,10.4));
#43507=CARTESIAN_POINT('Origin',(-57.,-82.5,28.825));
#43508=CARTESIAN_POINT('Origin',(-54.,-70.,19.8));
#43509=CARTESIAN_POINT('',(-54.,-57.,10.4));
#43510=CARTESIAN_POINT('',(-54.,-58.5,19.8));
#43511=CARTESIAN_POINT('',(-54.,-35.,28.825));
#43512=CARTESIAN_POINT('',(-54.,-79.,24.5));
#43513=CARTESIAN_POINT('Origin',(-54.,-79.,20.));
#43514=CARTESIAN_POINT('Origin',(-54.,-79.,20.));
#43515=CARTESIAN_POINT('',(-54.,-66.,25.));
#43516=CARTESIAN_POINT('Origin',(-54.,-66.,20.));
#43517=CARTESIAN_POINT('Origin',(-69.,-69.75,1.));
#43518=CARTESIAN_POINT('Origin',(39.,-43.,29.075));
#43519=CARTESIAN_POINT('',(42.,-43.,28.825));
#43520=CARTESIAN_POINT('Origin',(39.,-43.,28.825));
#43521=CARTESIAN_POINT('',(42.,-43.,28.825));
#43522=CARTESIAN_POINT('Origin',(42.25,-20.,29.075));
#43523=CARTESIAN_POINT('',(42.,-67.,28.825));
#43524=CARTESIAN_POINT('',(42.,-67.,28.825));
#43525=CARTESIAN_POINT('',(42.,-20.,28.825));
#43526=CARTESIAN_POINT('Origin',(45.,-67.,29.075));
#43527=CARTESIAN_POINT('',(45.,-70.,28.825));
#43528=CARTESIAN_POINT('Origin',(45.,-67.,28.825));
#43529=CARTESIAN_POINT('',(45.,-70.,28.825));
#43530=CARTESIAN_POINT('Origin',(21.,-69.75,29.075));
#43531=CARTESIAN_POINT('',(67.,-70.,28.825));
#43532=CARTESIAN_POINT('',(67.,-70.,28.825));
#43533=CARTESIAN_POINT('',(21.,-70.,28.825));
#43534=CARTESIAN_POINT('Origin',(67.,-67.,29.075));
#43535=CARTESIAN_POINT('',(70.,-67.,28.825));
#43536=CARTESIAN_POINT('Origin',(67.,-67.,28.825));
#43537=CARTESIAN_POINT('',(70.,-67.,28.825));
#43538=CARTESIAN_POINT('Origin',(69.75,-35.,29.075));
#43539=CARTESIAN_POINT('',(70.,67.,28.825));
#43540=CARTESIAN_POINT('',(70.,67.,28.825));
#43541=CARTESIAN_POINT('',(70.,-35.,28.825));
#43542=CARTESIAN_POINT('Origin',(67.,67.,29.075));
#43543=CARTESIAN_POINT('',(67.,70.,28.825));
#43544=CARTESIAN_POINT('Origin',(67.,67.,28.825));
#43545=CARTESIAN_POINT('',(67.,70.,28.825));
#43546=CARTESIAN_POINT('Origin',(35.,69.75,29.075));
#43547=CARTESIAN_POINT('',(-67.,70.,28.825));
#43548=CARTESIAN_POINT('',(-67.,70.,28.825));
#43549=CARTESIAN_POINT('',(35.,70.,28.825));
#43550=CARTESIAN_POINT('Origin',(-67.,67.,29.075));
#43551=CARTESIAN_POINT('',(-70.,67.,28.825));
#43552=CARTESIAN_POINT('Origin',(-67.,67.,28.825));
#43553=CARTESIAN_POINT('',(-70.,67.,28.825));
#43554=CARTESIAN_POINT('Origin',(-69.75,35.,29.075));
#43555=CARTESIAN_POINT('',(-70.,-51.,28.825));
#43556=CARTESIAN_POINT('',(-70.,-51.,28.825));
#43557=CARTESIAN_POINT('',(-70.,35.,28.825));
#43558=CARTESIAN_POINT('Origin',(-73.,-51.,29.075));
#43559=CARTESIAN_POINT('',(-73.,-54.,28.825));
#43560=CARTESIAN_POINT('Origin',(-73.,-51.,28.825));
#43561=CARTESIAN_POINT('',(-73.,-54.,28.825));
#43562=CARTESIAN_POINT('Origin',(-27.,-54.25,29.075));
#43563=CARTESIAN_POINT('',(-81.,-54.,28.825));
#43564=CARTESIAN_POINT('',(-81.,-54.,28.825));
#43565=CARTESIAN_POINT('',(-27.,-54.,28.825));
#43566=CARTESIAN_POINT('Origin',(-81.,-57.,29.075));
#43567=CARTESIAN_POINT('',(-84.,-57.,28.825));
#43568=CARTESIAN_POINT('Origin',(-81.,-57.,28.825));
#43569=CARTESIAN_POINT('',(-84.,-57.,28.825));
#43570=CARTESIAN_POINT('Origin',(-83.75,-27.,29.075));
#43571=CARTESIAN_POINT('',(-84.,-82.5,28.825));
#43572=CARTESIAN_POINT('',(-84.,-27.,28.825));
#43573=CARTESIAN_POINT('Origin',(-81.,-82.5,29.075));
#43574=CARTESIAN_POINT('',(-81.,-85.5,28.825));
#43575=CARTESIAN_POINT('Origin',(-42.,-85.25,29.075));
#43576=CARTESIAN_POINT('',(-57.,-85.5,28.825));
#43577=CARTESIAN_POINT('Origin',(-57.,-82.5,29.075));
#43578=CARTESIAN_POINT('',(-54.,-82.5,28.825));
#43579=CARTESIAN_POINT('Origin',(-54.25,-35.,29.075));
#43580=CARTESIAN_POINT('Origin',(-84.,-54.,1.));
#43581=CARTESIAN_POINT('',(-84.,-57.,1.));
#43582=CARTESIAN_POINT('Origin',(-81.,-57.,1.));
#43583=CARTESIAN_POINT('',(-81.,-54.,1.));
#43584=CARTESIAN_POINT('Origin',(-54.,-54.,1.));
#43585=CARTESIAN_POINT('',(-73.,-54.,10.4));
#43586=CARTESIAN_POINT('',(-57.,-54.,10.4));
#43587=CARTESIAN_POINT('Origin',(-73.,-51.,10.4));
#43588=CARTESIAN_POINT('',(-70.,-51.,10.4));
#43589=CARTESIAN_POINT('Origin',(-70.,70.,19.8));
#43590=CARTESIAN_POINT('',(-70.,67.,19.8));
#43591=CARTESIAN_POINT('Origin',(-67.,67.,19.8));
#43592=CARTESIAN_POINT('',(-67.,70.,19.8));
#43593=CARTESIAN_POINT('Origin',(70.,70.,19.8));
#43594=CARTESIAN_POINT('',(67.,70.,19.8));
#43595=CARTESIAN_POINT('Origin',(67.,67.,19.8));
#43596=CARTESIAN_POINT('',(70.,67.,19.8));
#43597=CARTESIAN_POINT('Origin',(70.,-70.,19.8));
#43598=CARTESIAN_POINT('',(70.,-67.,19.8));
#43599=CARTESIAN_POINT('Origin',(67.,-67.,19.8));
#43600=CARTESIAN_POINT('',(67.,-70.,19.8));
#43601=CARTESIAN_POINT('Origin',(42.,-70.,19.8));
#43602=CARTESIAN_POINT('',(45.,-70.,19.8));
#43603=CARTESIAN_POINT('Origin',(45.,-67.,19.8));
#43604=CARTESIAN_POINT('',(42.,-67.,19.8));
#43605=CARTESIAN_POINT('Origin',(42.,-40.,19.8));
#43606=CARTESIAN_POINT('',(42.,-43.,19.8));
#43607=CARTESIAN_POINT('Origin',(39.,-43.,19.8));
#43608=CARTESIAN_POINT('',(39.,-40.,19.8));
#43609=CARTESIAN_POINT('Origin',(-46.,-40.,19.8));
#43610=CARTESIAN_POINT('Origin',(37.5,0.,29.075));
#43611=CARTESIAN_POINT('',(25.25,-1.50019232895551E-15,29.075));
#43612=CARTESIAN_POINT('Origin',(-37.5,0.,29.075));
#43613=CARTESIAN_POINT('',(-49.75,-1.50019232895551E-15,29.075));
#43614=CARTESIAN_POINT('Origin',(0.,37.5,29.075));
#43615=CARTESIAN_POINT('',(-12.25,37.5,29.075));
#43616=CARTESIAN_POINT('Origin',(0.,0.,29.025));
#43617=CARTESIAN_POINT('',(-5.025,6.15385016571545E-16,28.725));
#43618=CARTESIAN_POINT('',(-5.325,-6.52124420545966E-16,29.025));
#43619=CARTESIAN_POINT('Origin',(0.,0.,28.725));
#43620=CARTESIAN_POINT('Origin',(0.,0.,29.325));
#43621=CARTESIAN_POINT('',(-5.025,6.15385016571545E-16,29.325));
#43622=CARTESIAN_POINT('Origin',(-60.,-79.,29.325));
#43623=CARTESIAN_POINT('',(-61.5,-79.,24.5));
#43624=CARTESIAN_POINT('',(-61.5,-79.,29.325));
#43625=CARTESIAN_POINT('',(-58.5,-79.,24.5));
#43626=CARTESIAN_POINT('Ctrl Pts',(-58.5,-79.,24.5));
#43627=CARTESIAN_POINT('Ctrl Pts',(-58.5,-78.810119017199,24.5));
#43628=CARTESIAN_POINT('Ctrl Pts',(-58.5382433687954,-78.6085507941687,
24.4868035691518));
#43629=CARTESIAN_POINT('Ctrl Pts',(-58.6917847708251,-78.2393832820639,
24.4391554329551));
#43630=CARTESIAN_POINT('Ctrl Pts',(-58.8070056851579,-78.0716739712825,
24.4053096652352));
#43631=CARTESIAN_POINT('Ctrl Pts',(-59.0717353764399,-77.8069442800004,
24.3411032840945));
#43632=CARTESIAN_POINT('Ctrl Pts',(-59.2394202300634,-77.6917706385605,
24.3063956191435));
#43633=CARTESIAN_POINT('Ctrl Pts',(-59.6084970398047,-77.5382644910968,
24.2567401743069));
#43634=CARTESIAN_POINT('Ctrl Pts',(-59.8100309093881,-77.5,24.2426406871193));
#43635=CARTESIAN_POINT('Ctrl Pts',(-60.1899690906119,-77.5,24.2426406871193));
#43636=CARTESIAN_POINT('Ctrl Pts',(-60.3915029601953,-77.5382644910968,
24.2567401743069));
#43637=CARTESIAN_POINT('Ctrl Pts',(-60.7605797699366,-77.6917706385605,
24.3063956191435));
#43638=CARTESIAN_POINT('Ctrl Pts',(-60.9282646235601,-77.8069442800004,
24.3411032840945));
#43639=CARTESIAN_POINT('Ctrl Pts',(-61.1929943148421,-78.0716739712825,
24.4053096652352));
#43640=CARTESIAN_POINT('Ctrl Pts',(-61.3082152291749,-78.2393832820639,
24.4391554329551));
#43641=CARTESIAN_POINT('Ctrl Pts',(-61.4617566312046,-78.6085507941687,
24.4868035691518));
#43642=CARTESIAN_POINT('Ctrl Pts',(-61.5,-78.810119017199,24.5));
#43643=CARTESIAN_POINT('Ctrl Pts',(-61.5,-79.,24.5));
#43644=CARTESIAN_POINT('',(-60.,-80.5,24.2426406871193));
#43645=CARTESIAN_POINT('Ctrl Pts',(-60.,-80.5,24.2426406871193));
#43646=CARTESIAN_POINT('Ctrl Pts',(-59.8100309093881,-80.5,24.2426406871193));
#43647=CARTESIAN_POINT('Ctrl Pts',(-59.6084970398047,-80.4617355089032,
24.2567401743069));
#43648=CARTESIAN_POINT('Ctrl Pts',(-59.2394202300634,-80.3082293614395,
24.3063956191435));
#43649=CARTESIAN_POINT('Ctrl Pts',(-59.0717353764399,-80.1930557199996,
24.3411032840945));
#43650=CARTESIAN_POINT('Ctrl Pts',(-58.8070056851579,-79.9283260287175,
24.4053096652352));
#43651=CARTESIAN_POINT('Ctrl Pts',(-58.6917847708251,-79.7606167179361,
24.4391554329551));
#43652=CARTESIAN_POINT('Ctrl Pts',(-58.5382433687954,-79.3914492058313,
24.4868035691518));
#43653=CARTESIAN_POINT('Ctrl Pts',(-58.5,-79.189880982801,24.5));
#43654=CARTESIAN_POINT('Ctrl Pts',(-58.5,-79.,24.5));
#43655=CARTESIAN_POINT('Ctrl Pts',(-61.5,-79.,24.5));
#43656=CARTESIAN_POINT('Ctrl Pts',(-61.5,-79.189880982801,24.5));
#43657=CARTESIAN_POINT('Ctrl Pts',(-61.4617566312046,-79.3914492058313,
24.4868035691518));
#43658=CARTESIAN_POINT('Ctrl Pts',(-61.3082152291749,-79.7606167179361,
24.4391554329551));
#43659=CARTESIAN_POINT('Ctrl Pts',(-61.1929943148421,-79.9283260287175,
24.4053096652352));
#43660=CARTESIAN_POINT('Ctrl Pts',(-60.9282646235601,-80.1930557199996,
24.3411032840945));
#43661=CARTESIAN_POINT('Ctrl Pts',(-60.7605797699366,-80.3082293614395,
24.3063956191435));
#43662=CARTESIAN_POINT('Ctrl Pts',(-60.3915029601953,-80.4617355089032,
24.2567401743069));
#43663=CARTESIAN_POINT('Ctrl Pts',(-60.1899690906119,-80.5,24.2426406871193));
#43664=CARTESIAN_POINT('Ctrl Pts',(-60.,-80.5,24.2426406871193));
#43665=CARTESIAN_POINT('Origin',(-60.,-79.,29.325));
#43666=CARTESIAN_POINT('',(-60.,-80.5,15.7573593128807));
#43667=CARTESIAN_POINT('',(-61.5,-79.,15.5));
#43668=CARTESIAN_POINT('Ctrl Pts',(-60.,-80.5,15.7573593128807));
#43669=CARTESIAN_POINT('Ctrl Pts',(-60.1899690906119,-80.5,15.7573593128807));
#43670=CARTESIAN_POINT('Ctrl Pts',(-60.3915029601953,-80.4617355089032,
15.7432598256931));
#43671=CARTESIAN_POINT('Ctrl Pts',(-60.7605797699366,-80.3082293614395,
15.6936043808565));
#43672=CARTESIAN_POINT('Ctrl Pts',(-60.9282646235601,-80.1930557199996,
15.6588967159055));
#43673=CARTESIAN_POINT('Ctrl Pts',(-61.1929943148421,-79.9283260287175,
15.5946903347648));
#43674=CARTESIAN_POINT('Ctrl Pts',(-61.3082152291749,-79.7606167179361,
15.5608445670449));
#43675=CARTESIAN_POINT('Ctrl Pts',(-61.4617566312046,-79.3914492058313,
15.5131964308482));
#43676=CARTESIAN_POINT('Ctrl Pts',(-61.5,-79.189880982801,15.5));
#43677=CARTESIAN_POINT('Ctrl Pts',(-61.5,-79.,15.5));
#43678=CARTESIAN_POINT('Ctrl Pts',(-61.5,-79.,15.5));
#43679=CARTESIAN_POINT('Ctrl Pts',(-61.5,-78.810119017199,15.5));
#43680=CARTESIAN_POINT('Ctrl Pts',(-61.4617566312046,-78.6085507941687,
15.5131964308482));
#43681=CARTESIAN_POINT('Ctrl Pts',(-61.3082152291749,-78.2393832820639,
15.5608445670449));
#43682=CARTESIAN_POINT('Ctrl Pts',(-61.1929943148421,-78.0716739712825,
15.5946903347648));
#43683=CARTESIAN_POINT('Ctrl Pts',(-60.9282646235601,-77.8069442800004,
15.6588967159055));
#43684=CARTESIAN_POINT('Ctrl Pts',(-60.7605797699366,-77.6917706385605,
15.6936043808565));
#43685=CARTESIAN_POINT('Ctrl Pts',(-60.3915029601953,-77.5382644910968,
15.7432598256931));
#43686=CARTESIAN_POINT('Ctrl Pts',(-60.1899690906119,-77.5,15.7573593128807));
#43687=CARTESIAN_POINT('Ctrl Pts',(-59.8100309093881,-77.5,15.7573593128807));
#43688=CARTESIAN_POINT('Ctrl Pts',(-59.6084970398047,-77.5382644910968,
15.7432598256931));
#43689=CARTESIAN_POINT('Ctrl Pts',(-59.2394202300634,-77.6917706385605,
15.6936043808565));
#43690=CARTESIAN_POINT('Ctrl Pts',(-59.0717353764399,-77.8069442800004,
15.6588967159055));
#43691=CARTESIAN_POINT('Ctrl Pts',(-58.8070056851579,-78.0716739712825,
15.5946903347648));
#43692=CARTESIAN_POINT('Ctrl Pts',(-58.6917847708251,-78.2393832820639,
15.5608445670449));
#43693=CARTESIAN_POINT('Ctrl Pts',(-58.5382433687954,-78.6085507941687,
15.5131964308482));
#43694=CARTESIAN_POINT('Ctrl Pts',(-58.5,-78.810119017199,15.5));
#43695=CARTESIAN_POINT('Ctrl Pts',(-58.5,-79.189880982801,15.5));
#43696=CARTESIAN_POINT('Ctrl Pts',(-58.5382433687954,-79.3914492058313,
15.5131964308482));
#43697=CARTESIAN_POINT('Ctrl Pts',(-58.6917847708251,-79.7606167179361,
15.5608445670449));
#43698=CARTESIAN_POINT('Ctrl Pts',(-58.8070056851579,-79.9283260287175,
15.5946903347648));
#43699=CARTESIAN_POINT('Ctrl Pts',(-59.0717353764399,-80.1930557199995,
15.6588967159055));
#43700=CARTESIAN_POINT('Ctrl Pts',(-59.2394202300634,-80.3082293614395,
15.6936043808565));
#43701=CARTESIAN_POINT('Ctrl Pts',(-59.6084970398047,-80.4617355089032,
15.7432598256931));
#43702=CARTESIAN_POINT('Ctrl Pts',(-59.8100309093881,-80.5,15.7573593128807));
#43703=CARTESIAN_POINT('Ctrl Pts',(-60.,-80.5,15.7573593128807));
#43704=CARTESIAN_POINT('',(-61.5,-79.,11.325));
#43705=CARTESIAN_POINT('',(-61.5,-79.,29.325));
#43706=CARTESIAN_POINT('Origin',(-60.,-79.,11.325));
#43707=CARTESIAN_POINT('Origin',(-60.,-79.,11.325));
#43708=CARTESIAN_POINT('Origin',(-54.,-79.,20.));
#43709=CARTESIAN_POINT('',(-54.,-79.,24.5));
#43710=CARTESIAN_POINT('',(-64.,-79.,24.5));
#43711=CARTESIAN_POINT('',(-54.,-79.,24.5));
#43712=CARTESIAN_POINT('Origin',(-64.,-79.,20.));
#43713=CARTESIAN_POINT('Origin',(-64.,-79.,20.));
#43714=CARTESIAN_POINT('Origin',(-54.,-66.,20.));
#43715=CARTESIAN_POINT('',(-58.5,-66.,25.));
#43716=CARTESIAN_POINT('',(-54.,-66.,25.));
#43717=CARTESIAN_POINT('Origin',(-58.5,-66.,20.));
#43718=CARTESIAN_POINT('Origin',(-58.5,-66.,20.));
#43719=CARTESIAN_POINT('Origin',(-18.75,56.25,20.825));
#43720=CARTESIAN_POINT('Origin',(-56.25,18.75,20.825));
#43721=CARTESIAN_POINT('Origin',(-52.425,52.425,29.325));
#43722=CARTESIAN_POINT('',(-56.6629,52.425,25.325));
#43723=CARTESIAN_POINT('',(-56.6629,52.425,29.325));
#43724=CARTESIAN_POINT('Origin',(-52.425,52.425,25.325));
#43725=CARTESIAN_POINT('Origin',(-52.425,52.425,25.325));
#43726=CARTESIAN_POINT('Origin',(-52.425,-52.425,29.325));
#43727=CARTESIAN_POINT('',(-57.425,-52.425,24.825));
#43728=CARTESIAN_POINT('',(-57.425,-52.425,29.325));
#43729=CARTESIAN_POINT('Origin',(-52.425,-52.425,24.825));
#43730=CARTESIAN_POINT('Origin',(-52.425,-52.425,24.825));
#43731=CARTESIAN_POINT('Origin',(52.425,52.425,29.325));
#43732=CARTESIAN_POINT('',(47.425,52.425,24.825));
#43733=CARTESIAN_POINT('',(47.425,52.425,29.325));
#43734=CARTESIAN_POINT('Origin',(52.425,52.425,24.825));
#43735=CARTESIAN_POINT('Origin',(52.425,52.425,24.825));
#43736=CARTESIAN_POINT('Origin',(-49.,-55.5,19.8));
#43737=CARTESIAN_POINT('',(-49.,-58.5,19.8));
#43738=CARTESIAN_POINT('Origin',(-54.,-58.5,19.8));
#43739=CARTESIAN_POINT('Origin',(-57.,-57.,10.4));
#82345=UNCERTAINTY_MEASURE_WITH_UNIT(LENGTH_MEASURE(0.01),#82385,
'DISTANCE_ACCURACY_VALUE',
'Maximum model space distance between geometric entities at asserted c
onnectivities');
#82363=UNCERTAINTY_MEASURE_WITH_UNIT(LENGTH_MEASURE(0.01),#82385,
'DISTANCE_ACCURACY_VALUE',
'Maximum model space distance between geometric entities at asserted c
onnectivities');
#82366=(
GEOMETRIC_REPRESENTATION_CONTEXT(3)
GLOBAL_UNCERTAINTY_ASSIGNED_CONTEXT((#82345))
GLOBAL_UNIT_ASSIGNED_CONTEXT((#82385,#82387,#82388))
REPRESENTATION_CONTEXT('','3D')
);
#82384=(
GEOMETRIC_REPRESENTATION_CONTEXT(3)
GLOBAL_UNCERTAINTY_ASSIGNED_CONTEXT((#82363))
GLOBAL_UNIT_ASSIGNED_CONTEXT((#82385,#82387,#82388))
REPRESENTATION_CONTEXT('','3D')
);
#82385=(
LENGTH_UNIT()
NAMED_UNIT(*)
SI_UNIT(.MILLI.,.METRE.)
);
#82387=(
NAMED_UNIT(*)
PLANE_ANGLE_UNIT()
SI_UNIT($,.RADIAN.)
);
#82388=(
NAMED_UNIT(*)
SI_UNIT($,.STERADIAN.)
SOLID_ANGLE_UNIT()
);
#82391=SHAPE_DEFINITION_REPRESENTATION(#82411,#82467);
#82411=PRODUCT_DEFINITION_SHAPE('',$,#82488);
#82467=SHAPE_REPRESENTATION('',(#31122),#82366);
#82485=PRODUCT_DEFINITION_CONTEXT('part definition',#82547,'design');
#82488=PRODUCT_DEFINITION('2026-10-20-12-38-05-983',
'02_Rotation_Carrier_Plate',#82508,#82485);
#82508=PRODUCT_DEFINITION_FORMATION('',$,#82551);
#82547=APPLICATION_CONTEXT(
'Core Data for Automotive Mechanical Design Process');
#82548=PRODUCT_CONTEXT('part definition',#82547,'mechanical');
#82551=PRODUCT('2026-10-20-12-38-05-983','02_Rotation_Carrier_Plate',$,
(#82548));
#82611=COLOUR_RGB('Light Blue',0.38,0.62,0.78);
#82612=FILL_AREA_STYLE_COLOUR('',#82611);
#82613=FILL_AREA_STYLE('',(#82612));
#82614=SURFACE_STYLE_FILL_AREA(#82613);
#82615=SURFACE_SIDE_STYLE('',(#82614));
#82616=SURFACE_STYLE_USAGE(.BOTH.,#82615);
#82617=PRESENTATION_STYLE_ASSIGNMENT((#82616));
ENDSEC;
END-ISO-10303-21;
